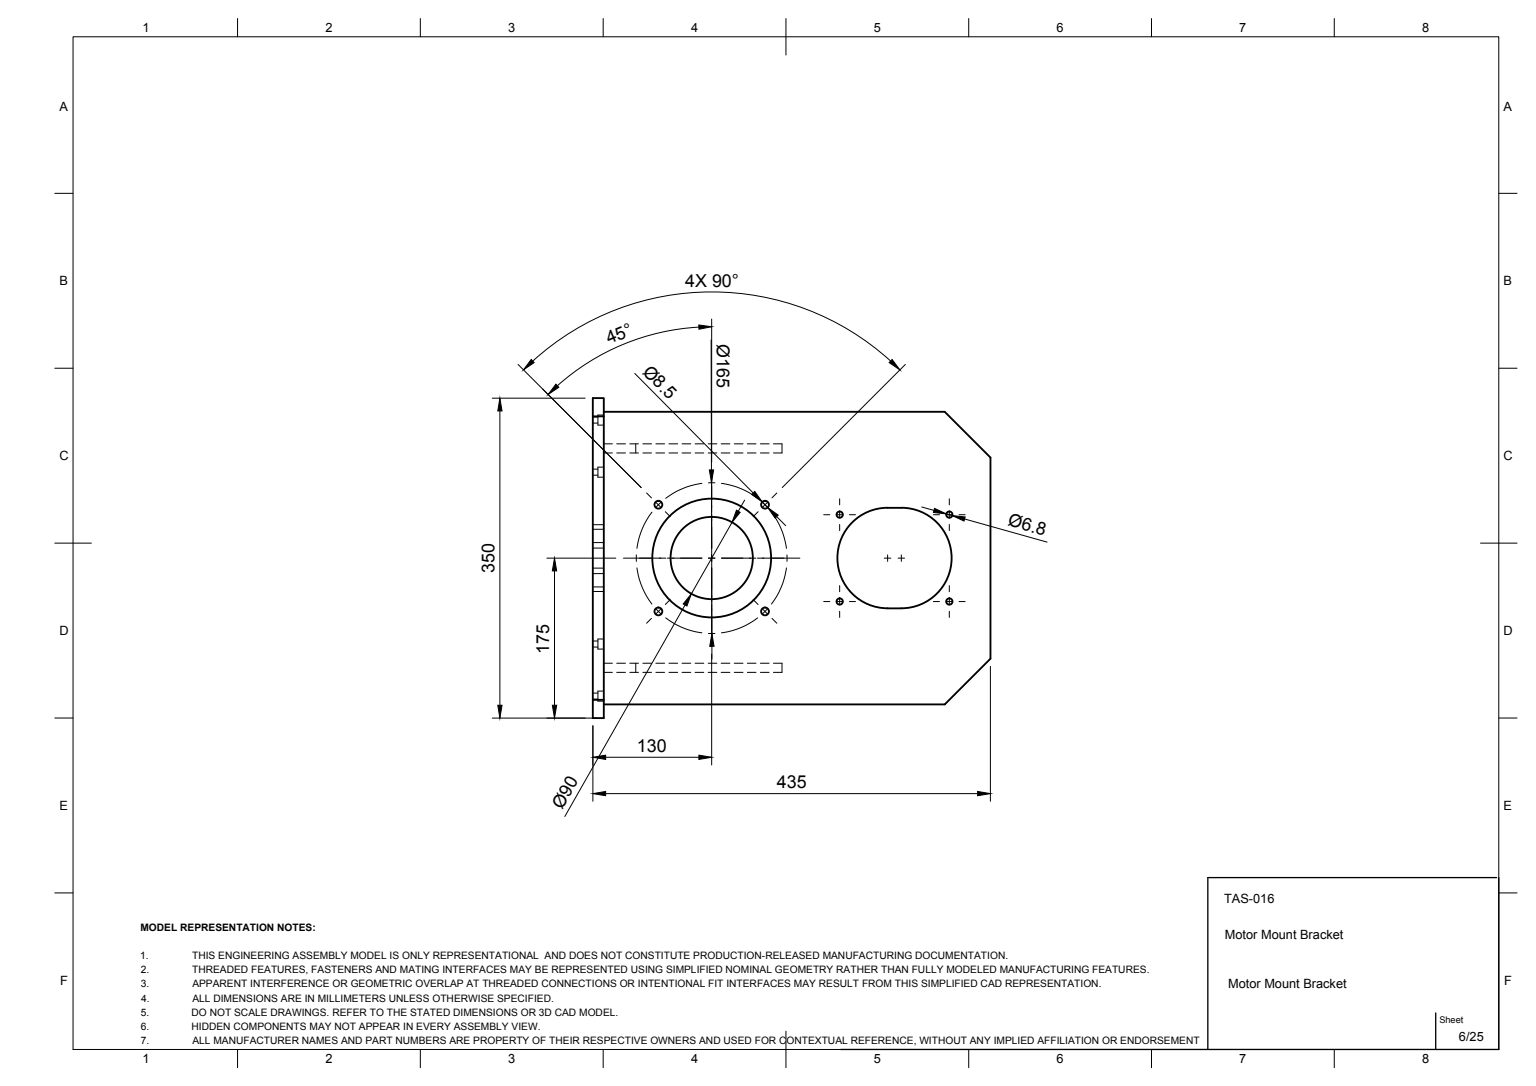
ISO-10303-21;
HEADER;
/* Generated by software containing ST-Developer
 * from STEP Tools, Inc. (www.steptools.com) 
 */

FILE_DESCRIPTION(
/* description */ ('STEP AP214'),
/* implementation_level */ '2;1');

FILE_NAME(
/* name */ 'Motor Mount Bracket.step',
/* time_stamp */ '2026-11-15T14:55:55-08:00',
/* author */ (''),
/* organization */ (''),
/* preprocessor_version */ 'ST-DEVELOPER v20.2',
/* originating_system */ 'Autodesk Translation Framework v15.17.0.0',
/* authorisation */ '');

FILE_SCHEMA (('AUTOMOTIVE_DESIGN { 1 0 10303 214 3 1 1 }'));
ENDSEC;

DATA;
#10=MECHANICAL_DESIGN_GEOMETRIC_PRESENTATION_REPRESENTATION('',(#947,#948,#949),#57079);
#887=SHAPE_REPRESENTATION_RELATIONSHIP('SRR','None',#57276,#916);
#916=ADVANCED_BREP_SHAPE_REPRESENTATION('',(#984,#985,#986),#57068);
#947=STYLED_ITEM('',(#57444),#984);
#948=STYLED_ITEM('',(#57444),#985);
#949=STYLED_ITEM('',(#57444),#986);
#984=MANIFOLD_SOLID_BREP('Body1',#24547);
#985=MANIFOLD_SOLID_BREP('Body2',#24548);
#986=MANIFOLD_SOLID_BREP('Body3',#24549);
#1195=FACE_BOUND('',#4460,.T.);
#1196=FACE_BOUND('',#4461,.T.);
#1197=FACE_BOUND('',#4462,.T.);
#1198=FACE_BOUND('',#4463,.T.);
#1199=FACE_BOUND('',#4464,.T.);
#1200=FACE_BOUND('',#4465,.T.);
#1201=FACE_BOUND('',#4466,.T.);
#1202=FACE_BOUND('',#4467,.T.);
#1203=FACE_BOUND('',#4468,.T.);
#1204=FACE_BOUND('',#4469,.T.);
#1205=FACE_BOUND('',#4470,.T.);
#1206=FACE_BOUND('',#4471,.T.);
#1207=FACE_BOUND('',#4472,.T.);
#1208=FACE_BOUND('',#4473,.T.);
#1209=FACE_BOUND('',#4474,.T.);
#1210=FACE_BOUND('',#4475,.T.);
#1211=FACE_BOUND('',#4476,.T.);
#1212=FACE_BOUND('',#4477,.T.);
#1213=FACE_BOUND('',#4478,.T.);
#1214=FACE_BOUND('',#4479,.T.);
#1215=FACE_BOUND('',#4480,.T.);
#1216=FACE_BOUND('',#4481,.T.);
#1217=FACE_BOUND('',#4486,.T.);
#1218=FACE_BOUND('',#4487,.T.);
#1219=FACE_BOUND('',#4488,.T.);
#1220=FACE_BOUND('',#4489,.T.);
#1221=FACE_BOUND('',#4490,.T.);
#1222=FACE_BOUND('',#4491,.T.);
#1223=FACE_BOUND('',#4492,.T.);
#1224=FACE_BOUND('',#4493,.T.);
#1225=FACE_BOUND('',#4494,.T.);
#1226=FACE_BOUND('',#4495,.T.);
#1227=FACE_BOUND('',#4497,.T.);
#1228=FACE_BOUND('',#4498,.T.);
#1229=FACE_BOUND('',#4499,.T.);
#1230=FACE_BOUND('',#4500,.T.);
#1231=FACE_BOUND('',#4501,.T.);
#1232=FACE_BOUND('',#4502,.T.);
#1233=FACE_BOUND('',#4503,.T.);
#1234=FACE_BOUND('',#4504,.T.);
#1235=FACE_BOUND('',#4505,.T.);
#1236=FACE_BOUND('',#4506,.T.);
#1237=FACE_BOUND('',#4508,.T.);
#1238=FACE_BOUND('',#4509,.T.);
#1239=FACE_BOUND('',#4510,.T.);
#1240=FACE_BOUND('',#4511,.T.);
#1241=FACE_BOUND('',#4512,.T.);
#1242=FACE_BOUND('',#4513,.T.);
#1243=FACE_BOUND('',#4514,.T.);
#1244=FACE_BOUND('',#4515,.T.);
#1245=FACE_BOUND('',#4516,.T.);
#1246=FACE_BOUND('',#4517,.T.);
#1247=FACE_BOUND('',#4518,.T.);
#1248=FACE_BOUND('',#4519,.T.);
#1249=FACE_BOUND('',#4520,.T.);
#1250=FACE_BOUND('',#4521,.T.);
#1251=FACE_BOUND('',#4522,.T.);
#1252=FACE_BOUND('',#4523,.T.);
#1253=FACE_BOUND('',#4524,.T.);
#1254=FACE_BOUND('',#4525,.T.);
#1255=FACE_BOUND('',#4526,.T.);
#1256=FACE_BOUND('',#4527,.T.);
#1257=FACE_BOUND('',#4528,.T.);
#1258=FACE_BOUND('',#4529,.T.);
#1259=FACE_BOUND('',#4530,.T.);
#1260=FACE_BOUND('',#4536,.T.);
#1261=FACE_BOUND('',#4538,.T.);
#1262=FACE_BOUND('',#4540,.T.);
#1263=FACE_BOUND('',#4542,.T.);
#1264=FACE_BOUND('',#4544,.T.);
#1265=FACE_BOUND('',#4546,.T.);
#1266=FACE_BOUND('',#4548,.T.);
#1267=FACE_BOUND('',#4550,.T.);
#1268=FACE_BOUND('',#4552,.T.);
#1269=FACE_BOUND('',#4554,.T.);
#1270=FACE_BOUND('',#4556,.T.);
#1271=FACE_BOUND('',#4558,.T.);
#1272=FACE_BOUND('',#4560,.T.);
#1273=FACE_BOUND('',#4562,.T.);
#1274=FACE_BOUND('',#4564,.T.);
#1275=FACE_BOUND('',#4566,.T.);
#1276=FACE_BOUND('',#4568,.T.);
#1680=PLANE('',#26069);
#1681=PLANE('',#26070);
#1682=PLANE('',#26071);
#1683=PLANE('',#26072);
#1684=PLANE('',#26073);
#1685=PLANE('',#26074);
#1686=PLANE('',#26075);
#1687=PLANE('',#26076);
#1688=PLANE('',#26077);
#1689=PLANE('',#26078);
#1690=PLANE('',#26079);
#1691=PLANE('',#26080);
#1692=PLANE('',#26081);
#1693=PLANE('',#26082);
#1694=PLANE('',#26230);
#1695=PLANE('',#26231);
#1696=PLANE('',#26232);
#1697=PLANE('',#26233);
#1698=PLANE('',#26234);
#1699=PLANE('',#26236);
#1700=PLANE('',#26238);
#1701=PLANE('',#26239);
#1702=PLANE('',#26240);
#1703=PLANE('',#26241);
#1704=PLANE('',#26242);
#1705=PLANE('',#26243);
#1706=PLANE('',#26244);
#1707=PLANE('',#26245);
#1708=PLANE('',#26246);
#1709=PLANE('',#26247);
#1710=PLANE('',#26248);
#1711=PLANE('',#26249);
#1712=PLANE('',#26250);
#1713=PLANE('',#26251);
#1714=PLANE('',#26252);
#1715=PLANE('',#26253);
#1716=PLANE('',#26254);
#1717=PLANE('',#26255);
#1718=PLANE('',#26256);
#1719=PLANE('',#26257);
#1720=PLANE('',#26258);
#1721=PLANE('',#26259);
#1722=PLANE('',#26260);
#1723=PLANE('',#26261);
#1724=PLANE('',#26262);
#1725=PLANE('',#26263);
#1726=PLANE('',#26265);
#1727=PLANE('',#26266);
#1728=PLANE('',#26267);
#1729=PLANE('',#26268);
#2826=FACE_OUTER_BOUND('',#4396,.T.);
#2827=FACE_OUTER_BOUND('',#4397,.T.);
#2828=FACE_OUTER_BOUND('',#4398,.T.);
#2829=FACE_OUTER_BOUND('',#4399,.T.);
#2830=FACE_OUTER_BOUND('',#4400,.T.);
#2831=FACE_OUTER_BOUND('',#4401,.T.);
#2832=FACE_OUTER_BOUND('',#4402,.T.);
#2833=FACE_OUTER_BOUND('',#4403,.T.);
#2834=FACE_OUTER_BOUND('',#4404,.T.);
#2835=FACE_OUTER_BOUND('',#4405,.T.);
#2836=FACE_OUTER_BOUND('',#4406,.T.);
#2837=FACE_OUTER_BOUND('',#4407,.T.);
#2838=FACE_OUTER_BOUND('',#4408,.T.);
#2839=FACE_OUTER_BOUND('',#4409,.T.);
#2840=FACE_OUTER_BOUND('',#4410,.T.);
#2841=FACE_OUTER_BOUND('',#4411,.T.);
#2842=FACE_OUTER_BOUND('',#4412,.T.);
#2843=FACE_OUTER_BOUND('',#4413,.T.);
#2844=FACE_OUTER_BOUND('',#4414,.T.);
#2845=FACE_OUTER_BOUND('',#4415,.T.);
#2846=FACE_OUTER_BOUND('',#4416,.T.);
#2847=FACE_OUTER_BOUND('',#4417,.T.);
#2848=FACE_OUTER_BOUND('',#4418,.T.);
#2849=FACE_OUTER_BOUND('',#4419,.T.);
#2850=FACE_OUTER_BOUND('',#4420,.T.);
#2851=FACE_OUTER_BOUND('',#4421,.T.);
#2852=FACE_OUTER_BOUND('',#4422,.T.);
#2853=FACE_OUTER_BOUND('',#4423,.T.);
#2854=FACE_OUTER_BOUND('',#4424,.T.);
#2855=FACE_OUTER_BOUND('',#4425,.T.);
#2856=FACE_OUTER_BOUND('',#4426,.T.);
#2857=FACE_OUTER_BOUND('',#4427,.T.);
#2858=FACE_OUTER_BOUND('',#4428,.T.);
#2859=FACE_OUTER_BOUND('',#4429,.T.);
#2860=FACE_OUTER_BOUND('',#4430,.T.);
#2861=FACE_OUTER_BOUND('',#4431,.T.);
#2862=FACE_OUTER_BOUND('',#4432,.T.);
#2863=FACE_OUTER_BOUND('',#4433,.T.);
#2864=FACE_OUTER_BOUND('',#4434,.T.);
#2865=FACE_OUTER_BOUND('',#4435,.T.);
#2866=FACE_OUTER_BOUND('',#4436,.T.);
#2867=FACE_OUTER_BOUND('',#4437,.T.);
#2868=FACE_OUTER_BOUND('',#4438,.T.);
#2869=FACE_OUTER_BOUND('',#4439,.T.);
#2870=FACE_OUTER_BOUND('',#4440,.T.);
#2871=FACE_OUTER_BOUND('',#4441,.T.);
#2872=FACE_OUTER_BOUND('',#4442,.T.);
#2873=FACE_OUTER_BOUND('',#4443,.T.);
#2874=FACE_OUTER_BOUND('',#4444,.T.);
#2875=FACE_OUTER_BOUND('',#4445,.T.);
#2876=FACE_OUTER_BOUND('',#4446,.T.);
#2877=FACE_OUTER_BOUND('',#4447,.T.);
#2878=FACE_OUTER_BOUND('',#4448,.T.);
#2879=FACE_OUTER_BOUND('',#4449,.T.);
#2880=FACE_OUTER_BOUND('',#4450,.T.);
#2881=FACE_OUTER_BOUND('',#4451,.T.);
#2882=FACE_OUTER_BOUND('',#4452,.T.);
#2883=FACE_OUTER_BOUND('',#4453,.T.);
#2884=FACE_OUTER_BOUND('',#4454,.T.);
#2885=FACE_OUTER_BOUND('',#4455,.T.);
#2886=FACE_OUTER_BOUND('',#4456,.T.);
#2887=FACE_OUTER_BOUND('',#4457,.T.);
#2888=FACE_OUTER_BOUND('',#4458,.T.);
#2889=FACE_OUTER_BOUND('',#4459,.T.);
#2890=FACE_OUTER_BOUND('',#4482,.T.);
#2891=FACE_OUTER_BOUND('',#4483,.T.);
#2892=FACE_OUTER_BOUND('',#4484,.T.);
#2893=FACE_OUTER_BOUND('',#4485,.T.);
#2894=FACE_OUTER_BOUND('',#4496,.T.);
#2895=FACE_OUTER_BOUND('',#4507,.T.);
#2896=FACE_OUTER_BOUND('',#4531,.T.);
#2897=FACE_OUTER_BOUND('',#4532,.T.);
#2898=FACE_OUTER_BOUND('',#4533,.T.);
#2899=FACE_OUTER_BOUND('',#4534,.T.);
#2900=FACE_OUTER_BOUND('',#4535,.T.);
#2901=FACE_OUTER_BOUND('',#4537,.T.);
#2902=FACE_OUTER_BOUND('',#4539,.T.);
#2903=FACE_OUTER_BOUND('',#4541,.T.);
#2904=FACE_OUTER_BOUND('',#4543,.T.);
#2905=FACE_OUTER_BOUND('',#4545,.T.);
#2906=FACE_OUTER_BOUND('',#4547,.T.);
#2907=FACE_OUTER_BOUND('',#4549,.T.);
#2908=FACE_OUTER_BOUND('',#4551,.T.);
#2909=FACE_OUTER_BOUND('',#4553,.T.);
#2910=FACE_OUTER_BOUND('',#4555,.T.);
#2911=FACE_OUTER_BOUND('',#4557,.T.);
#2912=FACE_OUTER_BOUND('',#4559,.T.);
#2913=FACE_OUTER_BOUND('',#4561,.T.);
#2914=FACE_OUTER_BOUND('',#4563,.T.);
#2915=FACE_OUTER_BOUND('',#4565,.T.);
#2916=FACE_OUTER_BOUND('',#4567,.T.);
#2917=FACE_OUTER_BOUND('',#4569,.T.);
#2918=FACE_OUTER_BOUND('',#4570,.T.);
#2919=FACE_OUTER_BOUND('',#4571,.T.);
#2920=FACE_OUTER_BOUND('',#4572,.T.);
#2921=FACE_OUTER_BOUND('',#4573,.T.);
#2922=FACE_OUTER_BOUND('',#4574,.T.);
#2923=FACE_OUTER_BOUND('',#4575,.T.);
#2924=FACE_OUTER_BOUND('',#4576,.T.);
#2925=FACE_OUTER_BOUND('',#4577,.T.);
#4396=EDGE_LOOP('',(#19072,#19073,#19074,#19075));
#4397=EDGE_LOOP('',(#19076,#19077,#19078,#19079));
#4398=EDGE_LOOP('',(#19080,#19081,#19082,#19083));
#4399=EDGE_LOOP('',(#19084,#19085,#19086,#19087));
#4400=EDGE_LOOP('',(#19088,#19089,#19090,#19091));
#4401=EDGE_LOOP('',(#19092,#19093,#19094,#19095,#19096));
#4402=EDGE_LOOP('',(#19097,#19098,#19099,#19100,#19101));
#4403=EDGE_LOOP('',(#19102,#19103,#19104,#19105));
#4404=EDGE_LOOP('',(#19106,#19107,#19108,#19109));
#4405=EDGE_LOOP('',(#19110,#19111,#19112,#19113));
#4406=EDGE_LOOP('',(#19114,#19115,#19116,#19117));
#4407=EDGE_LOOP('',(#19118,#19119,#19120,#19121));
#4408=EDGE_LOOP('',(#19122,#19123,#19124,#19125,#19126));
#4409=EDGE_LOOP('',(#19127,#19128,#19129,#19130,#19131));
#4410=EDGE_LOOP('',(#19132,#19133,#19134,#19135));
#4411=EDGE_LOOP('',(#19136,#19137,#19138,#19139));
#4412=EDGE_LOOP('',(#19140,#19141,#19142,#19143));
#4413=EDGE_LOOP('',(#19144,#19145,#19146,#19147));
#4414=EDGE_LOOP('',(#19148,#19149,#19150,#19151));
#4415=EDGE_LOOP('',(#19152,#19153,#19154,#19155));
#4416=EDGE_LOOP('',(#19156,#19157,#19158,#19159));
#4417=EDGE_LOOP('',(#19160,#19161,#19162,#19163));
#4418=EDGE_LOOP('',(#19164,#19165,#19166,#19167));
#4419=EDGE_LOOP('',(#19168,#19169,#19170,#19171));
#4420=EDGE_LOOP('',(#19172,#19173,#19174,#19175));
#4421=EDGE_LOOP('',(#19176,#19177,#19178,#19179));
#4422=EDGE_LOOP('',(#19180,#19181,#19182,#19183));
#4423=EDGE_LOOP('',(#19184,#19185,#19186,#19187));
#4424=EDGE_LOOP('',(#19188,#19189,#19190,#19191));
#4425=EDGE_LOOP('',(#19192,#19193,#19194,#19195));
#4426=EDGE_LOOP('',(#19196,#19197,#19198,#19199));
#4427=EDGE_LOOP('',(#19200,#19201,#19202,#19203));
#4428=EDGE_LOOP('',(#19204,#19205,#19206,#19207));
#4429=EDGE_LOOP('',(#19208,#19209,#19210,#19211));
#4430=EDGE_LOOP('',(#19212,#19213,#19214,#19215));
#4431=EDGE_LOOP('',(#19216,#19217,#19218,#19219));
#4432=EDGE_LOOP('',(#19220,#19221,#19222,#19223));
#4433=EDGE_LOOP('',(#19224,#19225,#19226,#19227));
#4434=EDGE_LOOP('',(#19228,#19229,#19230,#19231));
#4435=EDGE_LOOP('',(#19232,#19233,#19234,#19235));
#4436=EDGE_LOOP('',(#19236,#19237,#19238,#19239));
#4437=EDGE_LOOP('',(#19240,#19241,#19242,#19243));
#4438=EDGE_LOOP('',(#19244,#19245,#19246,#19247));
#4439=EDGE_LOOP('',(#19248,#19249,#19250,#19251));
#4440=EDGE_LOOP('',(#19252,#19253,#19254,#19255));
#4441=EDGE_LOOP('',(#19256,#19257,#19258,#19259));
#4442=EDGE_LOOP('',(#19260,#19261,#19262,#19263));
#4443=EDGE_LOOP('',(#19264,#19265,#19266,#19267));
#4444=EDGE_LOOP('',(#19268,#19269,#19270,#19271));
#4445=EDGE_LOOP('',(#19272,#19273,#19274,#19275));
#4446=EDGE_LOOP('',(#19276,#19277,#19278,#19279));
#4447=EDGE_LOOP('',(#19280,#19281,#19282,#19283));
#4448=EDGE_LOOP('',(#19284,#19285,#19286,#19287));
#4449=EDGE_LOOP('',(#19288,#19289,#19290,#19291));
#4450=EDGE_LOOP('',(#19292,#19293,#19294,#19295));
#4451=EDGE_LOOP('',(#19296,#19297,#19298,#19299));
#4452=EDGE_LOOP('',(#19300,#19301,#19302,#19303));
#4453=EDGE_LOOP('',(#19304,#19305,#19306,#19307));
#4454=EDGE_LOOP('',(#19308,#19309,#19310,#19311));
#4455=EDGE_LOOP('',(#19312,#19313,#19314,#19315));
#4456=EDGE_LOOP('',(#19316,#19317,#19318,#19319));
#4457=EDGE_LOOP('',(#19320,#19321,#19322,#19323));
#4458=EDGE_LOOP('',(#19324,#19325,#19326,#19327));
#4459=EDGE_LOOP('',(#19328,#19329,#19330,#19331,#19332,#19333,#19334,#19335));
#4460=EDGE_LOOP('',(#19336));
#4461=EDGE_LOOP('',(#19337));
#4462=EDGE_LOOP('',(#19338));
#4463=EDGE_LOOP('',(#19339));
#4464=EDGE_LOOP('',(#19340));
#4465=EDGE_LOOP('',(#19341));
#4466=EDGE_LOOP('',(#19342));
#4467=EDGE_LOOP('',(#19343));
#4468=EDGE_LOOP('',(#19344));
#4469=EDGE_LOOP('',(#19345));
#4470=EDGE_LOOP('',(#19346));
#4471=EDGE_LOOP('',(#19347));
#4472=EDGE_LOOP('',(#19348));
#4473=EDGE_LOOP('',(#19349));
#4474=EDGE_LOOP('',(#19350));
#4475=EDGE_LOOP('',(#19351));
#4476=EDGE_LOOP('',(#19352));
#4477=EDGE_LOOP('',(#19353));
#4478=EDGE_LOOP('',(#19354));
#4479=EDGE_LOOP('',(#19355));
#4480=EDGE_LOOP('',(#19356));
#4481=EDGE_LOOP('',(#19357));
#4482=EDGE_LOOP('',(#19358,#19359,#19360,#19361));
#4483=EDGE_LOOP('',(#19362,#19363,#19364,#19365));
#4484=EDGE_LOOP('',(#19366,#19367,#19368,#19369));
#4485=EDGE_LOOP('',(#19370,#19371,#19372,#19373,#19374,#19375));
#4486=EDGE_LOOP('',(#19376));
#4487=EDGE_LOOP('',(#19377));
#4488=EDGE_LOOP('',(#19378));
#4489=EDGE_LOOP('',(#19379));
#4490=EDGE_LOOP('',(#19380,#19381,#19382,#19383));
#4491=EDGE_LOOP('',(#19384));
#4492=EDGE_LOOP('',(#19385));
#4493=EDGE_LOOP('',(#19386));
#4494=EDGE_LOOP('',(#19387));
#4495=EDGE_LOOP('',(#19388));
#4496=EDGE_LOOP('',(#19389,#19390,#19391,#19392,#19393,#19394));
#4497=EDGE_LOOP('',(#19395,#19396,#19397,#19398));
#4498=EDGE_LOOP('',(#19399));
#4499=EDGE_LOOP('',(#19400));
#4500=EDGE_LOOP('',(#19401));
#4501=EDGE_LOOP('',(#19402));
#4502=EDGE_LOOP('',(#19403));
#4503=EDGE_LOOP('',(#19404));
#4504=EDGE_LOOP('',(#19405));
#4505=EDGE_LOOP('',(#19406));
#4506=EDGE_LOOP('',(#19407));
#4507=EDGE_LOOP('',(#19408,#19409,#19410,#19411,#19412,#19413,#19414,#19415));
#4508=EDGE_LOOP('',(#19416,#19417,#19418,#19419));
#4509=EDGE_LOOP('',(#19420));
#4510=EDGE_LOOP('',(#19421));
#4511=EDGE_LOOP('',(#19422));
#4512=EDGE_LOOP('',(#19423));
#4513=EDGE_LOOP('',(#19424));
#4514=EDGE_LOOP('',(#19425));
#4515=EDGE_LOOP('',(#19426));
#4516=EDGE_LOOP('',(#19427));
#4517=EDGE_LOOP('',(#19428));
#4518=EDGE_LOOP('',(#19429));
#4519=EDGE_LOOP('',(#19430));
#4520=EDGE_LOOP('',(#19431));
#4521=EDGE_LOOP('',(#19432));
#4522=EDGE_LOOP('',(#19433));
#4523=EDGE_LOOP('',(#19434));
#4524=EDGE_LOOP('',(#19435));
#4525=EDGE_LOOP('',(#19436));
#4526=EDGE_LOOP('',(#19437));
#4527=EDGE_LOOP('',(#19438));
#4528=EDGE_LOOP('',(#19439));
#4529=EDGE_LOOP('',(#19440));
#4530=EDGE_LOOP('',(#19441));
#4531=EDGE_LOOP('',(#19442,#19443,#19444,#19445));
#4532=EDGE_LOOP('',(#19446,#19447,#19448,#19449));
#4533=EDGE_LOOP('',(#19450,#19451,#19452,#19453));
#4534=EDGE_LOOP('',(#19454,#19455,#19456,#19457));
#4535=EDGE_LOOP('',(#19458));
#4536=EDGE_LOOP('',(#19459));
#4537=EDGE_LOOP('',(#19460));
#4538=EDGE_LOOP('',(#19461));
#4539=EDGE_LOOP('',(#19462));
#4540=EDGE_LOOP('',(#19463));
#4541=EDGE_LOOP('',(#19464));
#4542=EDGE_LOOP('',(#19465));
#4543=EDGE_LOOP('',(#19466));
#4544=EDGE_LOOP('',(#19467));
#4545=EDGE_LOOP('',(#19468));
#4546=EDGE_LOOP('',(#19469));
#4547=EDGE_LOOP('',(#19470));
#4548=EDGE_LOOP('',(#19471));
#4549=EDGE_LOOP('',(#19472));
#4550=EDGE_LOOP('',(#19473));
#4551=EDGE_LOOP('',(#19474));
#4552=EDGE_LOOP('',(#19475));
#4553=EDGE_LOOP('',(#19476));
#4554=EDGE_LOOP('',(#19477));
#4555=EDGE_LOOP('',(#19478));
#4556=EDGE_LOOP('',(#19479));
#4557=EDGE_LOOP('',(#19480));
#4558=EDGE_LOOP('',(#19481));
#4559=EDGE_LOOP('',(#19482));
#4560=EDGE_LOOP('',(#19483));
#4561=EDGE_LOOP('',(#19484));
#4562=EDGE_LOOP('',(#19485));
#4563=EDGE_LOOP('',(#19486));
#4564=EDGE_LOOP('',(#19487));
#4565=EDGE_LOOP('',(#19488));
#4566=EDGE_LOOP('',(#19489));
#4567=EDGE_LOOP('',(#19490));
#4568=EDGE_LOOP('',(#19491));
#4569=EDGE_LOOP('',(#19492,#19493,#19494,#19495));
#4570=EDGE_LOOP('',(#19496,#19497,#19498,#19499));
#4571=EDGE_LOOP('',(#19500,#19501,#19502,#19503));
#4572=EDGE_LOOP('',(#19504,#19505,#19506,#19507));
#4573=EDGE_LOOP('',(#19508,#19509,#19510,#19511));
#4574=EDGE_LOOP('',(#19512,#19513,#19514,#19515));
#4575=EDGE_LOOP('',(#19516,#19517,#19518,#19519));
#4576=EDGE_LOOP('',(#19520,#19521,#19522,#19523));
#4577=EDGE_LOOP('',(#19524,#19525,#19526,#19527));
#6035=LINE('',#52991,#8002);
#6036=LINE('',#52993,#8003);
#6037=LINE('',#52995,#8004);
#6038=LINE('',#52996,#8005);
#6039=LINE('',#52999,#8006);
#6040=LINE('',#53001,#8007);
#6041=LINE('',#53002,#8008);
#6042=LINE('',#53005,#8009);
#6043=LINE('',#53007,#8010);
#6044=LINE('',#53008,#8011);
#6045=LINE('',#53011,#8012);
#6046=LINE('',#53013,#8013);
#6047=LINE('',#53014,#8014);
#6048=LINE('',#53016,#8015);
#6049=LINE('',#53017,#8016);
#6050=LINE('',#53023,#8017);
#6051=LINE('',#53025,#8018);
#6052=LINE('',#53027,#8019);
#6053=LINE('',#53028,#8020);
#6054=LINE('',#53031,#8021);
#6055=LINE('',#53033,#8022);
#6056=LINE('',#53034,#8023);
#6057=LINE('',#53037,#8024);
#6058=LINE('',#53039,#8025);
#6059=LINE('',#53040,#8026);
#6060=LINE('',#53043,#8027);
#6061=LINE('',#53045,#8028);
#6062=LINE('',#53046,#8029);
#6063=LINE('',#53048,#8030);
#6064=LINE('',#53049,#8031);
#6065=LINE('',#53057,#8032);
#6066=LINE('',#53060,#8033);
#6067=LINE('',#53065,#8034);
#6068=LINE('',#53071,#8035);
#6069=LINE('',#53077,#8036);
#6070=LINE('',#53083,#8037);
#6071=LINE('',#53089,#8038);
#6072=LINE('',#53095,#8039);
#6073=LINE('',#53101,#8040);
#6074=LINE('',#53107,#8041);
#6075=LINE('',#53113,#8042);
#6076=LINE('',#53119,#8043);
#6077=LINE('',#53125,#8044);
#6078=LINE('',#53131,#8045);
#6079=LINE('',#53137,#8046);
#6080=LINE('',#53143,#8047);
#6081=LINE('',#53149,#8048);
#6082=LINE('',#53155,#8049);
#6083=LINE('',#53161,#8050);
#6084=LINE('',#53167,#8051);
#6085=LINE('',#53173,#8052);
#6086=LINE('',#53179,#8053);
#6087=LINE('',#53185,#8054);
#6088=LINE('',#53191,#8055);
#6089=LINE('',#53197,#8056);
#6090=LINE('',#53203,#8057);
#6091=LINE('',#53209,#8058);
#6092=LINE('',#53215,#8059);
#6093=LINE('',#53221,#8060);
#6094=LINE('',#53227,#8061);
#6095=LINE('',#53233,#8062);
#6096=LINE('',#53239,#8063);
#6097=LINE('',#53245,#8064);
#6098=LINE('',#53251,#8065);
#6099=LINE('',#53257,#8066);
#6100=LINE('',#53263,#8067);
#6101=LINE('',#53269,#8068);
#6102=LINE('',#53275,#8069);
#6103=LINE('',#53281,#8070);
#6104=LINE('',#53287,#8071);
#6105=LINE('',#53293,#8072);
#6106=LINE('',#53299,#8073);
#6107=LINE('',#53305,#8074);
#6108=LINE('',#53311,#8075);
#6109=LINE('',#53317,#8076);
#6110=LINE('',#53323,#8077);
#6111=LINE('',#53329,#8078);
#6112=LINE('',#53335,#8079);
#6113=LINE('',#53341,#8080);
#6114=LINE('',#53347,#8081);
#6115=LINE('',#53352,#8082);
#6116=LINE('',#53354,#8083);
#6117=LINE('',#53356,#8084);
#6118=LINE('',#53358,#8085);
#6119=LINE('',#53360,#8086);
#6120=LINE('',#53362,#8087);
#6121=LINE('',#53364,#8088);
#6122=LINE('',#53365,#8089);
#6123=LINE('',#53369,#8090);
#6124=LINE('',#53371,#8091);
#6125=LINE('',#53373,#8092);
#6126=LINE('',#53374,#8093);
#6127=LINE('',#53378,#8094);
#6128=LINE('',#53380,#8095);
#6129=LINE('',#53382,#8096);
#6130=LINE('',#53383,#8097);
#6131=LINE('',#53387,#8098);
#6132=LINE('',#53389,#8099);
#6133=LINE('',#53391,#8100);
#6134=LINE('',#53392,#8101);
#6135=LINE('',#53394,#8102);
#6136=LINE('',#53395,#8103);
#6137=LINE('',#53396,#8104);
#6138=LINE('',#53398,#8105);
#6139=LINE('',#53400,#8106);
#6140=LINE('',#53403,#8107);
#6141=LINE('',#53404,#8108);
#6142=LINE('',#53405,#8109);
#6143=LINE('',#53407,#8110);
#6144=LINE('',#53410,#8111);
#6145=LINE('',#53414,#8112);
#6146=LINE('',#53416,#8113);
#6147=LINE('',#53418,#8114);
#6148=LINE('',#53420,#8115);
#6149=LINE('',#53422,#8116);
#6150=LINE('',#53424,#8117);
#6151=LINE('',#53426,#8118);
#6152=LINE('',#53427,#8119);
#6153=LINE('',#53429,#8120);
#6154=LINE('',#53430,#8121);
#6155=LINE('',#53432,#8122);
#6156=LINE('',#53433,#8123);
#6157=LINE('',#53435,#8124);
#6158=LINE('',#53436,#8125);
#6159=LINE('',#53438,#8126);
#6160=LINE('',#53439,#8127);
#6161=LINE('',#53460,#8128);
#6162=LINE('',#53462,#8129);
#8002=VECTOR('',#30635,1000.);
#8003=VECTOR('',#30636,1000.);
#8004=VECTOR('',#30637,1000.);
#8005=VECTOR('',#30638,1000.);
#8006=VECTOR('',#30641,1000.);
#8007=VECTOR('',#30642,1000.);
#8008=VECTOR('',#30643,1000.);
#8009=VECTOR('',#30646,1000.);
#8010=VECTOR('',#30647,1000.);
#8011=VECTOR('',#30648,1000.);
#8012=VECTOR('',#30651,1000.);
#8013=VECTOR('',#30652,1000.);
#8014=VECTOR('',#30653,1000.);
#8015=VECTOR('',#30656,1000.);
#8016=VECTOR('',#30657,1000.);
#8017=VECTOR('',#30664,1000.);
#8018=VECTOR('',#30665,1000.);
#8019=VECTOR('',#30666,1000.);
#8020=VECTOR('',#30667,1000.);
#8021=VECTOR('',#30670,1000.);
#8022=VECTOR('',#30671,1000.);
#8023=VECTOR('',#30672,1000.);
#8024=VECTOR('',#30675,1000.);
#8025=VECTOR('',#30676,1000.);
#8026=VECTOR('',#30677,1000.);
#8027=VECTOR('',#30680,1000.);
#8028=VECTOR('',#30681,1000.);
#8029=VECTOR('',#30682,1000.);
#8030=VECTOR('',#30685,1000.);
#8031=VECTOR('',#30686,1000.);
#8032=VECTOR('',#30695,1000.);
#8033=VECTOR('',#30698,1000.);
#8034=VECTOR('',#30703,3.39999999999999);
#8035=VECTOR('',#30710,3.4);
#8036=VECTOR('',#30717,3.4);
#8037=VECTOR('',#30724,3.39999999999999);
#8038=VECTOR('',#30731,4.24999999999998);
#8039=VECTOR('',#30738,4.24999999999998);
#8040=VECTOR('',#30745,4.24999999999998);
#8041=VECTOR('',#30752,4.24999999999998);
#8042=VECTOR('',#30759,45.);
#8043=VECTOR('',#30766,65.);
#8044=VECTOR('',#30773,2.99999999999999);
#8045=VECTOR('',#30780,2.99999999999999);
#8046=VECTOR('',#30787,2.5);
#8047=VECTOR('',#30794,2.5);
#8048=VECTOR('',#30801,2.5);
#8049=VECTOR('',#30808,2.5);
#8050=VECTOR('',#30815,5.50000000000001);
#8051=VECTOR('',#30822,3.30000000000004);
#8052=VECTOR('',#30829,5.50000000000001);
#8053=VECTOR('',#30836,3.30000000000004);
#8054=VECTOR('',#30843,5.50000000000001);
#8055=VECTOR('',#30850,3.30000000000004);
#8056=VECTOR('',#30857,5.50000000000001);
#8057=VECTOR('',#30864,3.30000000000004);
#8058=VECTOR('',#30871,5.50000000000001);
#8059=VECTOR('',#30878,3.30000000000004);
#8060=VECTOR('',#30885,5.50000000000001);
#8061=VECTOR('',#30892,3.30000000000004);
#8062=VECTOR('',#30899,5.49999999999999);
#8063=VECTOR('',#30906,3.30000000000004);
#8064=VECTOR('',#30913,5.50000000000001);
#8065=VECTOR('',#30920,3.30000000000004);
#8066=VECTOR('',#30927,5.50000000000001);
#8067=VECTOR('',#30934,3.30000000000004);
#8068=VECTOR('',#30941,5.50000000000001);
#8069=VECTOR('',#30948,3.30000000000004);
#8070=VECTOR('',#30955,5.50000000000001);
#8071=VECTOR('',#30962,3.30000000000004);
#8072=VECTOR('',#30969,5.50000000000001);
#8073=VECTOR('',#30976,3.30000000000004);
#8074=VECTOR('',#30983,5.50000000000001);
#8075=VECTOR('',#30990,3.30000000000004);
#8076=VECTOR('',#30997,5.50000000000001);
#8077=VECTOR('',#31004,3.30000000000004);
#8078=VECTOR('',#31011,5.49999999999999);
#8079=VECTOR('',#31018,3.30000000000004);
#8080=VECTOR('',#31025,5.50000000000001);
#8081=VECTOR('',#31032,3.30000000000004);
#8082=VECTOR('',#31037,1000.);
#8083=VECTOR('',#31038,1000.);
#8084=VECTOR('',#31039,1000.);
#8085=VECTOR('',#31040,1000.);
#8086=VECTOR('',#31041,1000.);
#8087=VECTOR('',#31042,1000.);
#8088=VECTOR('',#31043,1000.);
#8089=VECTOR('',#31044,1000.);
#8090=VECTOR('',#31047,1000.);
#8091=VECTOR('',#31048,1000.);
#8092=VECTOR('',#31049,1000.);
#8093=VECTOR('',#31050,1000.);
#8094=VECTOR('',#31053,1000.);
#8095=VECTOR('',#31054,1000.);
#8096=VECTOR('',#31055,1000.);
#8097=VECTOR('',#31056,1000.);
#8098=VECTOR('',#31059,1000.);
#8099=VECTOR('',#31060,1000.);
#8100=VECTOR('',#31061,1000.);
#8101=VECTOR('',#31062,1000.);
#8102=VECTOR('',#31065,1000.);
#8103=VECTOR('',#31066,1000.);
#8104=VECTOR('',#31067,1000.);
#8105=VECTOR('',#31068,1000.);
#8106=VECTOR('',#31069,1000.);
#8107=VECTOR('',#31074,1000.);
#8108=VECTOR('',#31075,1000.);
#8109=VECTOR('',#31076,1000.);
#8110=VECTOR('',#31077,1000.);
#8111=VECTOR('',#31080,1000.);
#8112=VECTOR('',#31083,1000.);
#8113=VECTOR('',#31084,1000.);
#8114=VECTOR('',#31085,1000.);
#8115=VECTOR('',#31086,1000.);
#8116=VECTOR('',#31087,1000.);
#8117=VECTOR('',#31088,1000.);
#8118=VECTOR('',#31089,1000.);
#8119=VECTOR('',#31090,1000.);
#8120=VECTOR('',#31093,1000.);
#8121=VECTOR('',#31094,1000.);
#8122=VECTOR('',#31097,1000.);
#8123=VECTOR('',#31098,1000.);
#8124=VECTOR('',#31101,1000.);
#8125=VECTOR('',#31102,1000.);
#8126=VECTOR('',#31105,1000.);
#8127=VECTOR('',#31106,1000.);
#8128=VECTOR('',#31147,1000.);
#8129=VECTOR('',#31150,1000.);
#9708=CIRCLE('',#26084,55.);
#9709=CIRCLE('',#26085,55.);
#9710=CIRCLE('',#26087,3.39999999999999);
#9711=CIRCLE('',#26088,3.4);
#9712=CIRCLE('',#26090,3.4);
#9713=CIRCLE('',#26091,3.4);
#9714=CIRCLE('',#26093,3.4);
#9715=CIRCLE('',#26094,3.4);
#9716=CIRCLE('',#26096,3.39999999999999);
#9717=CIRCLE('',#26097,3.4);
#9718=CIRCLE('',#26099,4.24999999999998);
#9719=CIRCLE('',#26100,4.24999999999998);
#9720=CIRCLE('',#26102,4.24999999999998);
#9721=CIRCLE('',#26103,4.24999999999998);
#9722=CIRCLE('',#26105,4.24999999999998);
#9723=CIRCLE('',#26106,4.24999999999998);
#9724=CIRCLE('',#26108,4.24999999999998);
#9725=CIRCLE('',#26109,4.24999999999998);
#9726=CIRCLE('',#26111,45.);
#9727=CIRCLE('',#26112,45.);
#9728=CIRCLE('',#26114,65.);
#9729=CIRCLE('',#26115,65.);
#9730=CIRCLE('',#26117,2.99999999999999);
#9731=CIRCLE('',#26118,2.99999999999999);
#9732=CIRCLE('',#26120,2.99999999999999);
#9733=CIRCLE('',#26121,2.99999999999999);
#9734=CIRCLE('',#26123,2.5);
#9735=CIRCLE('',#26124,2.5);
#9736=CIRCLE('',#26126,2.5);
#9737=CIRCLE('',#26127,2.5);
#9738=CIRCLE('',#26129,2.5);
#9739=CIRCLE('',#26130,2.5);
#9740=CIRCLE('',#26132,2.5);
#9741=CIRCLE('',#26133,2.5);
#9742=CIRCLE('',#26135,5.50000000000001);
#9743=CIRCLE('',#26136,5.50000000000001);
#9744=CIRCLE('',#26138,3.30000000000008);
#9745=CIRCLE('',#26139,3.3);
#9746=CIRCLE('',#26141,5.50000000000001);
#9747=CIRCLE('',#26142,5.50000000000001);
#9748=CIRCLE('',#26144,3.30000000000008);
#9749=CIRCLE('',#26145,3.3);
#9750=CIRCLE('',#26147,5.50000000000001);
#9751=CIRCLE('',#26148,5.50000000000001);
#9752=CIRCLE('',#26150,3.30000000000008);
#9753=CIRCLE('',#26151,3.3);
#9754=CIRCLE('',#26153,5.50000000000001);
#9755=CIRCLE('',#26154,5.50000000000001);
#9756=CIRCLE('',#26156,3.30000000000008);
#9757=CIRCLE('',#26157,3.3);
#9758=CIRCLE('',#26159,5.50000000000001);
#9759=CIRCLE('',#26160,5.50000000000001);
#9760=CIRCLE('',#26162,3.30000000000008);
#9761=CIRCLE('',#26163,3.3);
#9762=CIRCLE('',#26165,5.50000000000001);
#9763=CIRCLE('',#26166,5.50000000000001);
#9764=CIRCLE('',#26168,3.30000000000008);
#9765=CIRCLE('',#26169,3.3);
#9766=CIRCLE('',#26171,5.49999999999999);
#9767=CIRCLE('',#26172,5.49999999999999);
#9768=CIRCLE('',#26174,3.30000000000008);
#9769=CIRCLE('',#26175,3.3);
#9770=CIRCLE('',#26177,5.50000000000001);
#9771=CIRCLE('',#26178,5.50000000000001);
#9772=CIRCLE('',#26180,3.30000000000008);
#9773=CIRCLE('',#26181,3.3);
#9774=CIRCLE('',#26183,5.50000000000001);
#9775=CIRCLE('',#26184,5.50000000000001);
#9776=CIRCLE('',#26186,3.30000000000008);
#9777=CIRCLE('',#26187,3.3);
#9778=CIRCLE('',#26189,5.50000000000001);
#9779=CIRCLE('',#26190,5.50000000000001);
#9780=CIRCLE('',#26192,3.30000000000008);
#9781=CIRCLE('',#26193,3.3);
#9782=CIRCLE('',#26195,5.50000000000001);
#9783=CIRCLE('',#26196,5.50000000000001);
#9784=CIRCLE('',#26198,3.30000000000008);
#9785=CIRCLE('',#26199,3.3);
#9786=CIRCLE('',#26201,5.50000000000001);
#9787=CIRCLE('',#26202,5.50000000000001);
#9788=CIRCLE('',#26204,3.30000000000008);
#9789=CIRCLE('',#26205,3.3);
#9790=CIRCLE('',#26207,5.50000000000001);
#9791=CIRCLE('',#26208,5.50000000000001);
#9792=CIRCLE('',#26210,3.30000000000008);
#9793=CIRCLE('',#26211,3.3);
#9794=CIRCLE('',#26213,5.50000000000001);
#9795=CIRCLE('',#26214,5.50000000000001);
#9796=CIRCLE('',#26216,3.30000000000008);
#9797=CIRCLE('',#26217,3.3);
#9798=CIRCLE('',#26219,5.49999999999999);
#9799=CIRCLE('',#26220,5.49999999999999);
#9800=CIRCLE('',#26222,3.30000000000008);
#9801=CIRCLE('',#26223,3.3);
#9802=CIRCLE('',#26225,5.50000000000001);
#9803=CIRCLE('',#26226,5.50000000000001);
#9804=CIRCLE('',#26228,3.30000000000008);
#9805=CIRCLE('',#26229,3.3);
#9806=CIRCLE('',#26235,55.);
#9807=CIRCLE('',#26237,55.);
#11289=VERTEX_POINT('',#52989);
#11290=VERTEX_POINT('',#52990);
#11291=VERTEX_POINT('',#52992);
#11292=VERTEX_POINT('',#52994);
#11293=VERTEX_POINT('',#52998);
#11294=VERTEX_POINT('',#53000);
#11295=VERTEX_POINT('',#53004);
#11296=VERTEX_POINT('',#53006);
#11297=VERTEX_POINT('',#53010);
#11298=VERTEX_POINT('',#53012);
#11299=VERTEX_POINT('',#53021);
#11300=VERTEX_POINT('',#53022);
#11301=VERTEX_POINT('',#53024);
#11302=VERTEX_POINT('',#53026);
#11303=VERTEX_POINT('',#53030);
#11304=VERTEX_POINT('',#53032);
#11305=VERTEX_POINT('',#53036);
#11306=VERTEX_POINT('',#53038);
#11307=VERTEX_POINT('',#53042);
#11308=VERTEX_POINT('',#53044);
#11309=VERTEX_POINT('',#53053);
#11310=VERTEX_POINT('',#53054);
#11311=VERTEX_POINT('',#53056);
#11312=VERTEX_POINT('',#53058);
#11313=VERTEX_POINT('',#53062);
#11314=VERTEX_POINT('',#53064);
#11315=VERTEX_POINT('',#53068);
#11316=VERTEX_POINT('',#53070);
#11317=VERTEX_POINT('',#53074);
#11318=VERTEX_POINT('',#53076);
#11319=VERTEX_POINT('',#53080);
#11320=VERTEX_POINT('',#53082);
#11321=VERTEX_POINT('',#53086);
#11322=VERTEX_POINT('',#53088);
#11323=VERTEX_POINT('',#53092);
#11324=VERTEX_POINT('',#53094);
#11325=VERTEX_POINT('',#53098);
#11326=VERTEX_POINT('',#53100);
#11327=VERTEX_POINT('',#53104);
#11328=VERTEX_POINT('',#53106);
#11329=VERTEX_POINT('',#53110);
#11330=VERTEX_POINT('',#53112);
#11331=VERTEX_POINT('',#53116);
#11332=VERTEX_POINT('',#53118);
#11333=VERTEX_POINT('',#53122);
#11334=VERTEX_POINT('',#53124);
#11335=VERTEX_POINT('',#53128);
#11336=VERTEX_POINT('',#53130);
#11337=VERTEX_POINT('',#53134);
#11338=VERTEX_POINT('',#53136);
#11339=VERTEX_POINT('',#53140);
#11340=VERTEX_POINT('',#53142);
#11341=VERTEX_POINT('',#53146);
#11342=VERTEX_POINT('',#53148);
#11343=VERTEX_POINT('',#53152);
#11344=VERTEX_POINT('',#53154);
#11345=VERTEX_POINT('',#53158);
#11346=VERTEX_POINT('',#53160);
#11347=VERTEX_POINT('',#53164);
#11348=VERTEX_POINT('',#53166);
#11349=VERTEX_POINT('',#53170);
#11350=VERTEX_POINT('',#53172);
#11351=VERTEX_POINT('',#53176);
#11352=VERTEX_POINT('',#53178);
#11353=VERTEX_POINT('',#53182);
#11354=VERTEX_POINT('',#53184);
#11355=VERTEX_POINT('',#53188);
#11356=VERTEX_POINT('',#53190);
#11357=VERTEX_POINT('',#53194);
#11358=VERTEX_POINT('',#53196);
#11359=VERTEX_POINT('',#53200);
#11360=VERTEX_POINT('',#53202);
#11361=VERTEX_POINT('',#53206);
#11362=VERTEX_POINT('',#53208);
#11363=VERTEX_POINT('',#53212);
#11364=VERTEX_POINT('',#53214);
#11365=VERTEX_POINT('',#53218);
#11366=VERTEX_POINT('',#53220);
#11367=VERTEX_POINT('',#53224);
#11368=VERTEX_POINT('',#53226);
#11369=VERTEX_POINT('',#53230);
#11370=VERTEX_POINT('',#53232);
#11371=VERTEX_POINT('',#53236);
#11372=VERTEX_POINT('',#53238);
#11373=VERTEX_POINT('',#53242);
#11374=VERTEX_POINT('',#53244);
#11375=VERTEX_POINT('',#53248);
#11376=VERTEX_POINT('',#53250);
#11377=VERTEX_POINT('',#53254);
#11378=VERTEX_POINT('',#53256);
#11379=VERTEX_POINT('',#53260);
#11380=VERTEX_POINT('',#53262);
#11381=VERTEX_POINT('',#53266);
#11382=VERTEX_POINT('',#53268);
#11383=VERTEX_POINT('',#53272);
#11384=VERTEX_POINT('',#53274);
#11385=VERTEX_POINT('',#53278);
#11386=VERTEX_POINT('',#53280);
#11387=VERTEX_POINT('',#53284);
#11388=VERTEX_POINT('',#53286);
#11389=VERTEX_POINT('',#53290);
#11390=VERTEX_POINT('',#53292);
#11391=VERTEX_POINT('',#53296);
#11392=VERTEX_POINT('',#53298);
#11393=VERTEX_POINT('',#53302);
#11394=VERTEX_POINT('',#53304);
#11395=VERTEX_POINT('',#53308);
#11396=VERTEX_POINT('',#53310);
#11397=VERTEX_POINT('',#53314);
#11398=VERTEX_POINT('',#53316);
#11399=VERTEX_POINT('',#53320);
#11400=VERTEX_POINT('',#53322);
#11401=VERTEX_POINT('',#53326);
#11402=VERTEX_POINT('',#53328);
#11403=VERTEX_POINT('',#53332);
#11404=VERTEX_POINT('',#53334);
#11405=VERTEX_POINT('',#53338);
#11406=VERTEX_POINT('',#53340);
#11407=VERTEX_POINT('',#53344);
#11408=VERTEX_POINT('',#53346);
#11409=VERTEX_POINT('',#53350);
#11410=VERTEX_POINT('',#53351);
#11411=VERTEX_POINT('',#53353);
#11412=VERTEX_POINT('',#53355);
#11413=VERTEX_POINT('',#53357);
#11414=VERTEX_POINT('',#53359);
#11415=VERTEX_POINT('',#53361);
#11416=VERTEX_POINT('',#53363);
#11417=VERTEX_POINT('',#53367);
#11418=VERTEX_POINT('',#53368);
#11419=VERTEX_POINT('',#53370);
#11420=VERTEX_POINT('',#53372);
#11421=VERTEX_POINT('',#53376);
#11422=VERTEX_POINT('',#53377);
#11423=VERTEX_POINT('',#53379);
#11424=VERTEX_POINT('',#53381);
#11425=VERTEX_POINT('',#53385);
#11426=VERTEX_POINT('',#53386);
#11427=VERTEX_POINT('',#53388);
#11428=VERTEX_POINT('',#53390);
#11429=VERTEX_POINT('',#53397);
#11430=VERTEX_POINT('',#53399);
#11431=VERTEX_POINT('',#53406);
#11432=VERTEX_POINT('',#53408);
#11433=VERTEX_POINT('',#53412);
#11434=VERTEX_POINT('',#53413);
#11435=VERTEX_POINT('',#53415);
#11436=VERTEX_POINT('',#53417);
#11437=VERTEX_POINT('',#53419);
#11438=VERTEX_POINT('',#53421);
#11439=VERTEX_POINT('',#53423);
#11440=VERTEX_POINT('',#53425);
#14081=EDGE_CURVE('',#11289,#11290,#6035,.T.);
#14082=EDGE_CURVE('',#11291,#11289,#6036,.T.);
#14083=EDGE_CURVE('',#11291,#11292,#6037,.T.);
#14084=EDGE_CURVE('',#11292,#11290,#6038,.T.);
#14085=EDGE_CURVE('',#11293,#11289,#6039,.T.);
#14086=EDGE_CURVE('',#11294,#11293,#6040,.T.);
#14087=EDGE_CURVE('',#11294,#11291,#6041,.T.);
#14088=EDGE_CURVE('',#11295,#11293,#6042,.T.);
#14089=EDGE_CURVE('',#11296,#11295,#6043,.T.);
#14090=EDGE_CURVE('',#11296,#11294,#6044,.T.);
#14091=EDGE_CURVE('',#11295,#11297,#6045,.T.);
#14092=EDGE_CURVE('',#11298,#11297,#6046,.T.);
#14093=EDGE_CURVE('',#11296,#11298,#6047,.T.);
#14094=EDGE_CURVE('',#11297,#11290,#6048,.T.);
#14095=EDGE_CURVE('',#11298,#11292,#6049,.T.);
#14096=EDGE_CURVE('',#11299,#11300,#6050,.T.);
#14097=EDGE_CURVE('',#11301,#11300,#6051,.T.);
#14098=EDGE_CURVE('',#11302,#11301,#6052,.T.);
#14099=EDGE_CURVE('',#11302,#11299,#6053,.T.);
#14100=EDGE_CURVE('',#11303,#11299,#6054,.T.);
#14101=EDGE_CURVE('',#11304,#11302,#6055,.T.);
#14102=EDGE_CURVE('',#11304,#11303,#6056,.T.);
#14103=EDGE_CURVE('',#11305,#11303,#6057,.T.);
#14104=EDGE_CURVE('',#11306,#11304,#6058,.T.);
#14105=EDGE_CURVE('',#11306,#11305,#6059,.T.);
#14106=EDGE_CURVE('',#11305,#11307,#6060,.T.);
#14107=EDGE_CURVE('',#11306,#11308,#6061,.T.);
#14108=EDGE_CURVE('',#11308,#11307,#6062,.T.);
#14109=EDGE_CURVE('',#11307,#11300,#6063,.T.);
#14110=EDGE_CURVE('',#11308,#11301,#6064,.T.);
#14111=EDGE_CURVE('',#11309,#11310,#9708,.T.);
#14112=EDGE_CURVE('',#11310,#11311,#6065,.T.);
#14113=EDGE_CURVE('',#11311,#11312,#9709,.T.);
#14114=EDGE_CURVE('',#11309,#11312,#6066,.T.);
#14115=EDGE_CURVE('',#11313,#11313,#9710,.T.);
#14116=EDGE_CURVE('',#11313,#11314,#6067,.T.);
#14117=EDGE_CURVE('',#11314,#11314,#9711,.T.);
#14118=EDGE_CURVE('',#11315,#11315,#9712,.T.);
#14119=EDGE_CURVE('',#11315,#11316,#6068,.T.);
#14120=EDGE_CURVE('',#11316,#11316,#9713,.T.);
#14121=EDGE_CURVE('',#11317,#11317,#9714,.T.);
#14122=EDGE_CURVE('',#11317,#11318,#6069,.T.);
#14123=EDGE_CURVE('',#11318,#11318,#9715,.T.);
#14124=EDGE_CURVE('',#11319,#11319,#9716,.T.);
#14125=EDGE_CURVE('',#11319,#11320,#6070,.T.);
#14126=EDGE_CURVE('',#11320,#11320,#9717,.T.);
#14127=EDGE_CURVE('',#11321,#11321,#9718,.T.);
#14128=EDGE_CURVE('',#11321,#11322,#6071,.T.);
#14129=EDGE_CURVE('',#11322,#11322,#9719,.T.);
#14130=EDGE_CURVE('',#11323,#11323,#9720,.T.);
#14131=EDGE_CURVE('',#11323,#11324,#6072,.T.);
#14132=EDGE_CURVE('',#11324,#11324,#9721,.T.);
#14133=EDGE_CURVE('',#11325,#11325,#9722,.T.);
#14134=EDGE_CURVE('',#11325,#11326,#6073,.T.);
#14135=EDGE_CURVE('',#11326,#11326,#9723,.T.);
#14136=EDGE_CURVE('',#11327,#11327,#9724,.T.);
#14137=EDGE_CURVE('',#11327,#11328,#6074,.T.);
#14138=EDGE_CURVE('',#11328,#11328,#9725,.T.);
#14139=EDGE_CURVE('',#11329,#11329,#9726,.T.);
#14140=EDGE_CURVE('',#11329,#11330,#6075,.T.);
#14141=EDGE_CURVE('',#11330,#11330,#9727,.T.);
#14142=EDGE_CURVE('',#11331,#11331,#9728,.T.);
#14143=EDGE_CURVE('',#11331,#11332,#6076,.T.);
#14144=EDGE_CURVE('',#11332,#11332,#9729,.T.);
#14145=EDGE_CURVE('',#11333,#11333,#9730,.T.);
#14146=EDGE_CURVE('',#11333,#11334,#6077,.T.);
#14147=EDGE_CURVE('',#11334,#11334,#9731,.T.);
#14148=EDGE_CURVE('',#11335,#11335,#9732,.T.);
#14149=EDGE_CURVE('',#11335,#11336,#6078,.T.);
#14150=EDGE_CURVE('',#11336,#11336,#9733,.T.);
#14151=EDGE_CURVE('',#11337,#11337,#9734,.T.);
#14152=EDGE_CURVE('',#11337,#11338,#6079,.T.);
#14153=EDGE_CURVE('',#11338,#11338,#9735,.T.);
#14154=EDGE_CURVE('',#11339,#11339,#9736,.T.);
#14155=EDGE_CURVE('',#11339,#11340,#6080,.T.);
#14156=EDGE_CURVE('',#11340,#11340,#9737,.T.);
#14157=EDGE_CURVE('',#11341,#11341,#9738,.T.);
#14158=EDGE_CURVE('',#11341,#11342,#6081,.T.);
#14159=EDGE_CURVE('',#11342,#11342,#9739,.T.);
#14160=EDGE_CURVE('',#11343,#11343,#9740,.T.);
#14161=EDGE_CURVE('',#11343,#11344,#6082,.T.);
#14162=EDGE_CURVE('',#11344,#11344,#9741,.T.);
#14163=EDGE_CURVE('',#11345,#11345,#9742,.T.);
#14164=EDGE_CURVE('',#11345,#11346,#6083,.T.);
#14165=EDGE_CURVE('',#11346,#11346,#9743,.T.);
#14166=EDGE_CURVE('',#11347,#11347,#9744,.T.);
#14167=EDGE_CURVE('',#11347,#11348,#6084,.T.);
#14168=EDGE_CURVE('',#11348,#11348,#9745,.T.);
#14169=EDGE_CURVE('',#11349,#11349,#9746,.T.);
#14170=EDGE_CURVE('',#11349,#11350,#6085,.T.);
#14171=EDGE_CURVE('',#11350,#11350,#9747,.T.);
#14172=EDGE_CURVE('',#11351,#11351,#9748,.T.);
#14173=EDGE_CURVE('',#11351,#11352,#6086,.T.);
#14174=EDGE_CURVE('',#11352,#11352,#9749,.T.);
#14175=EDGE_CURVE('',#11353,#11353,#9750,.T.);
#14176=EDGE_CURVE('',#11353,#11354,#6087,.T.);
#14177=EDGE_CURVE('',#11354,#11354,#9751,.T.);
#14178=EDGE_CURVE('',#11355,#11355,#9752,.T.);
#14179=EDGE_CURVE('',#11355,#11356,#6088,.T.);
#14180=EDGE_CURVE('',#11356,#11356,#9753,.T.);
#14181=EDGE_CURVE('',#11357,#11357,#9754,.T.);
#14182=EDGE_CURVE('',#11357,#11358,#6089,.T.);
#14183=EDGE_CURVE('',#11358,#11358,#9755,.T.);
#14184=EDGE_CURVE('',#11359,#11359,#9756,.T.);
#14185=EDGE_CURVE('',#11359,#11360,#6090,.T.);
#14186=EDGE_CURVE('',#11360,#11360,#9757,.T.);
#14187=EDGE_CURVE('',#11361,#11361,#9758,.T.);
#14188=EDGE_CURVE('',#11361,#11362,#6091,.T.);
#14189=EDGE_CURVE('',#11362,#11362,#9759,.T.);
#14190=EDGE_CURVE('',#11363,#11363,#9760,.T.);
#14191=EDGE_CURVE('',#11363,#11364,#6092,.T.);
#14192=EDGE_CURVE('',#11364,#11364,#9761,.T.);
#14193=EDGE_CURVE('',#11365,#11365,#9762,.T.);
#14194=EDGE_CURVE('',#11365,#11366,#6093,.T.);
#14195=EDGE_CURVE('',#11366,#11366,#9763,.T.);
#14196=EDGE_CURVE('',#11367,#11367,#9764,.T.);
#14197=EDGE_CURVE('',#11367,#11368,#6094,.T.);
#14198=EDGE_CURVE('',#11368,#11368,#9765,.T.);
#14199=EDGE_CURVE('',#11369,#11369,#9766,.T.);
#14200=EDGE_CURVE('',#11369,#11370,#6095,.T.);
#14201=EDGE_CURVE('',#11370,#11370,#9767,.T.);
#14202=EDGE_CURVE('',#11371,#11371,#9768,.T.);
#14203=EDGE_CURVE('',#11371,#11372,#6096,.T.);
#14204=EDGE_CURVE('',#11372,#11372,#9769,.T.);
#14205=EDGE_CURVE('',#11373,#11373,#9770,.T.);
#14206=EDGE_CURVE('',#11373,#11374,#6097,.T.);
#14207=EDGE_CURVE('',#11374,#11374,#9771,.T.);
#14208=EDGE_CURVE('',#11375,#11375,#9772,.T.);
#14209=EDGE_CURVE('',#11375,#11376,#6098,.T.);
#14210=EDGE_CURVE('',#11376,#11376,#9773,.T.);
#14211=EDGE_CURVE('',#11377,#11377,#9774,.T.);
#14212=EDGE_CURVE('',#11377,#11378,#6099,.T.);
#14213=EDGE_CURVE('',#11378,#11378,#9775,.T.);
#14214=EDGE_CURVE('',#11379,#11379,#9776,.T.);
#14215=EDGE_CURVE('',#11379,#11380,#6100,.T.);
#14216=EDGE_CURVE('',#11380,#11380,#9777,.T.);
#14217=EDGE_CURVE('',#11381,#11381,#9778,.T.);
#14218=EDGE_CURVE('',#11381,#11382,#6101,.T.);
#14219=EDGE_CURVE('',#11382,#11382,#9779,.T.);
#14220=EDGE_CURVE('',#11383,#11383,#9780,.T.);
#14221=EDGE_CURVE('',#11383,#11384,#6102,.T.);
#14222=EDGE_CURVE('',#11384,#11384,#9781,.T.);
#14223=EDGE_CURVE('',#11385,#11385,#9782,.T.);
#14224=EDGE_CURVE('',#11385,#11386,#6103,.T.);
#14225=EDGE_CURVE('',#11386,#11386,#9783,.T.);
#14226=EDGE_CURVE('',#11387,#11387,#9784,.T.);
#14227=EDGE_CURVE('',#11387,#11388,#6104,.T.);
#14228=EDGE_CURVE('',#11388,#11388,#9785,.T.);
#14229=EDGE_CURVE('',#11389,#11389,#9786,.T.);
#14230=EDGE_CURVE('',#11389,#11390,#6105,.T.);
#14231=EDGE_CURVE('',#11390,#11390,#9787,.T.);
#14232=EDGE_CURVE('',#11391,#11391,#9788,.T.);
#14233=EDGE_CURVE('',#11391,#11392,#6106,.T.);
#14234=EDGE_CURVE('',#11392,#11392,#9789,.T.);
#14235=EDGE_CURVE('',#11393,#11393,#9790,.T.);
#14236=EDGE_CURVE('',#11393,#11394,#6107,.T.);
#14237=EDGE_CURVE('',#11394,#11394,#9791,.T.);
#14238=EDGE_CURVE('',#11395,#11395,#9792,.T.);
#14239=EDGE_CURVE('',#11395,#11396,#6108,.T.);
#14240=EDGE_CURVE('',#11396,#11396,#9793,.T.);
#14241=EDGE_CURVE('',#11397,#11397,#9794,.T.);
#14242=EDGE_CURVE('',#11397,#11398,#6109,.T.);
#14243=EDGE_CURVE('',#11398,#11398,#9795,.T.);
#14244=EDGE_CURVE('',#11399,#11399,#9796,.T.);
#14245=EDGE_CURVE('',#11399,#11400,#6110,.T.);
#14246=EDGE_CURVE('',#11400,#11400,#9797,.T.);
#14247=EDGE_CURVE('',#11401,#11401,#9798,.T.);
#14248=EDGE_CURVE('',#11401,#11402,#6111,.T.);
#14249=EDGE_CURVE('',#11402,#11402,#9799,.T.);
#14250=EDGE_CURVE('',#11403,#11403,#9800,.T.);
#14251=EDGE_CURVE('',#11403,#11404,#6112,.T.);
#14252=EDGE_CURVE('',#11404,#11404,#9801,.T.);
#14253=EDGE_CURVE('',#11405,#11405,#9802,.T.);
#14254=EDGE_CURVE('',#11405,#11406,#6113,.T.);
#14255=EDGE_CURVE('',#11406,#11406,#9803,.T.);
#14256=EDGE_CURVE('',#11407,#11407,#9804,.T.);
#14257=EDGE_CURVE('',#11407,#11408,#6114,.T.);
#14258=EDGE_CURVE('',#11408,#11408,#9805,.T.);
#14259=EDGE_CURVE('',#11409,#11410,#6115,.T.);
#14260=EDGE_CURVE('',#11409,#11411,#6116,.T.);
#14261=EDGE_CURVE('',#11412,#11411,#6117,.T.);
#14262=EDGE_CURVE('',#11412,#11413,#6118,.T.);
#14263=EDGE_CURVE('',#11414,#11413,#6119,.T.);
#14264=EDGE_CURVE('',#11414,#11415,#6120,.T.);
#14265=EDGE_CURVE('',#11416,#11415,#6121,.T.);
#14266=EDGE_CURVE('',#11416,#11410,#6122,.T.);
#14267=EDGE_CURVE('',#11417,#11418,#6123,.T.);
#14268=EDGE_CURVE('',#11418,#11419,#6124,.T.);
#14269=EDGE_CURVE('',#11420,#11419,#6125,.T.);
#14270=EDGE_CURVE('',#11420,#11417,#6126,.T.);
#14271=EDGE_CURVE('',#11421,#11422,#6127,.T.);
#14272=EDGE_CURVE('',#11421,#11423,#6128,.T.);
#14273=EDGE_CURVE('',#11423,#11424,#6129,.T.);
#14274=EDGE_CURVE('',#11424,#11422,#6130,.T.);
#14275=EDGE_CURVE('',#11425,#11426,#6131,.T.);
#14276=EDGE_CURVE('',#11426,#11427,#6132,.T.);
#14277=EDGE_CURVE('',#11428,#11427,#6133,.T.);
#14278=EDGE_CURVE('',#11425,#11428,#6134,.T.);
#14279=EDGE_CURVE('',#11419,#11421,#6135,.T.);
#14280=EDGE_CURVE('',#11422,#11426,#6136,.T.);
#14281=EDGE_CURVE('',#11425,#11420,#6137,.T.);
#14282=EDGE_CURVE('',#11310,#11429,#6138,.T.);
#14283=EDGE_CURVE('',#11430,#11309,#6139,.T.);
#14284=EDGE_CURVE('',#11429,#11430,#9806,.T.);
#14285=EDGE_CURVE('',#11423,#11418,#6140,.T.);
#14286=EDGE_CURVE('',#11428,#11417,#6141,.T.);
#14287=EDGE_CURVE('',#11427,#11424,#6142,.T.);
#14288=EDGE_CURVE('',#11431,#11311,#6143,.T.);
#14289=EDGE_CURVE('',#11432,#11431,#9807,.T.);
#14290=EDGE_CURVE('',#11312,#11432,#6144,.T.);
#14291=EDGE_CURVE('',#11433,#11434,#6145,.T.);
#14292=EDGE_CURVE('',#11434,#11435,#6146,.T.);
#14293=EDGE_CURVE('',#11435,#11436,#6147,.T.);
#14294=EDGE_CURVE('',#11436,#11437,#6148,.T.);
#14295=EDGE_CURVE('',#11437,#11438,#6149,.T.);
#14296=EDGE_CURVE('',#11438,#11439,#6150,.T.);
#14297=EDGE_CURVE('',#11439,#11440,#6151,.T.);
#14298=EDGE_CURVE('',#11440,#11433,#6152,.T.);
#14299=EDGE_CURVE('',#11435,#11409,#6153,.T.);
#14300=EDGE_CURVE('',#11410,#11436,#6154,.T.);
#14301=EDGE_CURVE('',#11415,#11438,#6155,.T.);
#14302=EDGE_CURVE('',#11437,#11416,#6156,.T.);
#14303=EDGE_CURVE('',#11413,#11440,#6157,.T.);
#14304=EDGE_CURVE('',#11439,#11414,#6158,.T.);
#14305=EDGE_CURVE('',#11411,#11434,#6159,.T.);
#14306=EDGE_CURVE('',#11433,#11412,#6160,.T.);
#14307=EDGE_CURVE('',#11429,#11431,#6161,.T.);
#14308=EDGE_CURVE('',#11430,#11432,#6162,.T.);
#19072=ORIENTED_EDGE('',*,*,#14081,.F.);
#19073=ORIENTED_EDGE('',*,*,#14082,.F.);
#19074=ORIENTED_EDGE('',*,*,#14083,.T.);
#19075=ORIENTED_EDGE('',*,*,#14084,.T.);
#19076=ORIENTED_EDGE('',*,*,#14085,.F.);
#19077=ORIENTED_EDGE('',*,*,#14086,.F.);
#19078=ORIENTED_EDGE('',*,*,#14087,.T.);
#19079=ORIENTED_EDGE('',*,*,#14082,.T.);
#19080=ORIENTED_EDGE('',*,*,#14088,.F.);
#19081=ORIENTED_EDGE('',*,*,#14089,.F.);
#19082=ORIENTED_EDGE('',*,*,#14090,.T.);
#19083=ORIENTED_EDGE('',*,*,#14086,.T.);
#19084=ORIENTED_EDGE('',*,*,#14091,.T.);
#19085=ORIENTED_EDGE('',*,*,#14092,.F.);
#19086=ORIENTED_EDGE('',*,*,#14093,.F.);
#19087=ORIENTED_EDGE('',*,*,#14089,.T.);
#19088=ORIENTED_EDGE('',*,*,#14094,.T.);
#19089=ORIENTED_EDGE('',*,*,#14084,.F.);
#19090=ORIENTED_EDGE('',*,*,#14095,.F.);
#19091=ORIENTED_EDGE('',*,*,#14092,.T.);
#19092=ORIENTED_EDGE('',*,*,#14083,.F.);
#19093=ORIENTED_EDGE('',*,*,#14087,.F.);
#19094=ORIENTED_EDGE('',*,*,#14090,.F.);
#19095=ORIENTED_EDGE('',*,*,#14093,.T.);
#19096=ORIENTED_EDGE('',*,*,#14095,.T.);
#19097=ORIENTED_EDGE('',*,*,#14081,.T.);
#19098=ORIENTED_EDGE('',*,*,#14094,.F.);
#19099=ORIENTED_EDGE('',*,*,#14091,.F.);
#19100=ORIENTED_EDGE('',*,*,#14088,.T.);
#19101=ORIENTED_EDGE('',*,*,#14085,.T.);
#19102=ORIENTED_EDGE('',*,*,#14096,.T.);
#19103=ORIENTED_EDGE('',*,*,#14097,.F.);
#19104=ORIENTED_EDGE('',*,*,#14098,.F.);
#19105=ORIENTED_EDGE('',*,*,#14099,.T.);
#19106=ORIENTED_EDGE('',*,*,#14100,.T.);
#19107=ORIENTED_EDGE('',*,*,#14099,.F.);
#19108=ORIENTED_EDGE('',*,*,#14101,.F.);
#19109=ORIENTED_EDGE('',*,*,#14102,.T.);
#19110=ORIENTED_EDGE('',*,*,#14103,.T.);
#19111=ORIENTED_EDGE('',*,*,#14102,.F.);
#19112=ORIENTED_EDGE('',*,*,#14104,.F.);
#19113=ORIENTED_EDGE('',*,*,#14105,.T.);
#19114=ORIENTED_EDGE('',*,*,#14106,.F.);
#19115=ORIENTED_EDGE('',*,*,#14105,.F.);
#19116=ORIENTED_EDGE('',*,*,#14107,.T.);
#19117=ORIENTED_EDGE('',*,*,#14108,.T.);
#19118=ORIENTED_EDGE('',*,*,#14109,.F.);
#19119=ORIENTED_EDGE('',*,*,#14108,.F.);
#19120=ORIENTED_EDGE('',*,*,#14110,.T.);
#19121=ORIENTED_EDGE('',*,*,#14097,.T.);
#19122=ORIENTED_EDGE('',*,*,#14098,.T.);
#19123=ORIENTED_EDGE('',*,*,#14110,.F.);
#19124=ORIENTED_EDGE('',*,*,#14107,.F.);
#19125=ORIENTED_EDGE('',*,*,#14104,.T.);
#19126=ORIENTED_EDGE('',*,*,#14101,.T.);
#19127=ORIENTED_EDGE('',*,*,#14096,.F.);
#19128=ORIENTED_EDGE('',*,*,#14100,.F.);
#19129=ORIENTED_EDGE('',*,*,#14103,.F.);
#19130=ORIENTED_EDGE('',*,*,#14106,.T.);
#19131=ORIENTED_EDGE('',*,*,#14109,.T.);
#19132=ORIENTED_EDGE('',*,*,#14111,.T.);
#19133=ORIENTED_EDGE('',*,*,#14112,.T.);
#19134=ORIENTED_EDGE('',*,*,#14113,.T.);
#19135=ORIENTED_EDGE('',*,*,#14114,.F.);
#19136=ORIENTED_EDGE('',*,*,#14115,.T.);
#19137=ORIENTED_EDGE('',*,*,#14116,.T.);
#19138=ORIENTED_EDGE('',*,*,#14117,.T.);
#19139=ORIENTED_EDGE('',*,*,#14116,.F.);
#19140=ORIENTED_EDGE('',*,*,#14118,.T.);
#19141=ORIENTED_EDGE('',*,*,#14119,.T.);
#19142=ORIENTED_EDGE('',*,*,#14120,.T.);
#19143=ORIENTED_EDGE('',*,*,#14119,.F.);
#19144=ORIENTED_EDGE('',*,*,#14121,.T.);
#19145=ORIENTED_EDGE('',*,*,#14122,.T.);
#19146=ORIENTED_EDGE('',*,*,#14123,.T.);
#19147=ORIENTED_EDGE('',*,*,#14122,.F.);
#19148=ORIENTED_EDGE('',*,*,#14124,.T.);
#19149=ORIENTED_EDGE('',*,*,#14125,.T.);
#19150=ORIENTED_EDGE('',*,*,#14126,.T.);
#19151=ORIENTED_EDGE('',*,*,#14125,.F.);
#19152=ORIENTED_EDGE('',*,*,#14127,.T.);
#19153=ORIENTED_EDGE('',*,*,#14128,.T.);
#19154=ORIENTED_EDGE('',*,*,#14129,.T.);
#19155=ORIENTED_EDGE('',*,*,#14128,.F.);
#19156=ORIENTED_EDGE('',*,*,#14130,.T.);
#19157=ORIENTED_EDGE('',*,*,#14131,.T.);
#19158=ORIENTED_EDGE('',*,*,#14132,.T.);
#19159=ORIENTED_EDGE('',*,*,#14131,.F.);
#19160=ORIENTED_EDGE('',*,*,#14133,.T.);
#19161=ORIENTED_EDGE('',*,*,#14134,.T.);
#19162=ORIENTED_EDGE('',*,*,#14135,.T.);
#19163=ORIENTED_EDGE('',*,*,#14134,.F.);
#19164=ORIENTED_EDGE('',*,*,#14136,.T.);
#19165=ORIENTED_EDGE('',*,*,#14137,.T.);
#19166=ORIENTED_EDGE('',*,*,#14138,.T.);
#19167=ORIENTED_EDGE('',*,*,#14137,.F.);
#19168=ORIENTED_EDGE('',*,*,#14139,.T.);
#19169=ORIENTED_EDGE('',*,*,#14140,.T.);
#19170=ORIENTED_EDGE('',*,*,#14141,.T.);
#19171=ORIENTED_EDGE('',*,*,#14140,.F.);
#19172=ORIENTED_EDGE('',*,*,#14142,.F.);
#19173=ORIENTED_EDGE('',*,*,#14143,.T.);
#19174=ORIENTED_EDGE('',*,*,#14144,.T.);
#19175=ORIENTED_EDGE('',*,*,#14143,.F.);
#19176=ORIENTED_EDGE('',*,*,#14145,.T.);
#19177=ORIENTED_EDGE('',*,*,#14146,.T.);
#19178=ORIENTED_EDGE('',*,*,#14147,.T.);
#19179=ORIENTED_EDGE('',*,*,#14146,.F.);
#19180=ORIENTED_EDGE('',*,*,#14148,.T.);
#19181=ORIENTED_EDGE('',*,*,#14149,.T.);
#19182=ORIENTED_EDGE('',*,*,#14150,.T.);
#19183=ORIENTED_EDGE('',*,*,#14149,.F.);
#19184=ORIENTED_EDGE('',*,*,#14151,.T.);
#19185=ORIENTED_EDGE('',*,*,#14152,.T.);
#19186=ORIENTED_EDGE('',*,*,#14153,.T.);
#19187=ORIENTED_EDGE('',*,*,#14152,.F.);
#19188=ORIENTED_EDGE('',*,*,#14154,.T.);
#19189=ORIENTED_EDGE('',*,*,#14155,.T.);
#19190=ORIENTED_EDGE('',*,*,#14156,.T.);
#19191=ORIENTED_EDGE('',*,*,#14155,.F.);
#19192=ORIENTED_EDGE('',*,*,#14157,.T.);
#19193=ORIENTED_EDGE('',*,*,#14158,.T.);
#19194=ORIENTED_EDGE('',*,*,#14159,.T.);
#19195=ORIENTED_EDGE('',*,*,#14158,.F.);
#19196=ORIENTED_EDGE('',*,*,#14160,.T.);
#19197=ORIENTED_EDGE('',*,*,#14161,.T.);
#19198=ORIENTED_EDGE('',*,*,#14162,.T.);
#19199=ORIENTED_EDGE('',*,*,#14161,.F.);
#19200=ORIENTED_EDGE('',*,*,#14163,.F.);
#19201=ORIENTED_EDGE('',*,*,#14164,.T.);
#19202=ORIENTED_EDGE('',*,*,#14165,.T.);
#19203=ORIENTED_EDGE('',*,*,#14164,.F.);
#19204=ORIENTED_EDGE('',*,*,#14166,.F.);
#19205=ORIENTED_EDGE('',*,*,#14167,.T.);
#19206=ORIENTED_EDGE('',*,*,#14168,.T.);
#19207=ORIENTED_EDGE('',*,*,#14167,.F.);
#19208=ORIENTED_EDGE('',*,*,#14169,.F.);
#19209=ORIENTED_EDGE('',*,*,#14170,.T.);
#19210=ORIENTED_EDGE('',*,*,#14171,.T.);
#19211=ORIENTED_EDGE('',*,*,#14170,.F.);
#19212=ORIENTED_EDGE('',*,*,#14172,.F.);
#19213=ORIENTED_EDGE('',*,*,#14173,.T.);
#19214=ORIENTED_EDGE('',*,*,#14174,.T.);
#19215=ORIENTED_EDGE('',*,*,#14173,.F.);
#19216=ORIENTED_EDGE('',*,*,#14175,.F.);
#19217=ORIENTED_EDGE('',*,*,#14176,.T.);
#19218=ORIENTED_EDGE('',*,*,#14177,.T.);
#19219=ORIENTED_EDGE('',*,*,#14176,.F.);
#19220=ORIENTED_EDGE('',*,*,#14178,.F.);
#19221=ORIENTED_EDGE('',*,*,#14179,.T.);
#19222=ORIENTED_EDGE('',*,*,#14180,.T.);
#19223=ORIENTED_EDGE('',*,*,#14179,.F.);
#19224=ORIENTED_EDGE('',*,*,#14181,.F.);
#19225=ORIENTED_EDGE('',*,*,#14182,.T.);
#19226=ORIENTED_EDGE('',*,*,#14183,.T.);
#19227=ORIENTED_EDGE('',*,*,#14182,.F.);
#19228=ORIENTED_EDGE('',*,*,#14184,.F.);
#19229=ORIENTED_EDGE('',*,*,#14185,.T.);
#19230=ORIENTED_EDGE('',*,*,#14186,.T.);
#19231=ORIENTED_EDGE('',*,*,#14185,.F.);
#19232=ORIENTED_EDGE('',*,*,#14187,.F.);
#19233=ORIENTED_EDGE('',*,*,#14188,.T.);
#19234=ORIENTED_EDGE('',*,*,#14189,.T.);
#19235=ORIENTED_EDGE('',*,*,#14188,.F.);
#19236=ORIENTED_EDGE('',*,*,#14190,.F.);
#19237=ORIENTED_EDGE('',*,*,#14191,.T.);
#19238=ORIENTED_EDGE('',*,*,#14192,.T.);
#19239=ORIENTED_EDGE('',*,*,#14191,.F.);
#19240=ORIENTED_EDGE('',*,*,#14193,.F.);
#19241=ORIENTED_EDGE('',*,*,#14194,.T.);
#19242=ORIENTED_EDGE('',*,*,#14195,.T.);
#19243=ORIENTED_EDGE('',*,*,#14194,.F.);
#19244=ORIENTED_EDGE('',*,*,#14196,.F.);
#19245=ORIENTED_EDGE('',*,*,#14197,.T.);
#19246=ORIENTED_EDGE('',*,*,#14198,.T.);
#19247=ORIENTED_EDGE('',*,*,#14197,.F.);
#19248=ORIENTED_EDGE('',*,*,#14199,.F.);
#19249=ORIENTED_EDGE('',*,*,#14200,.T.);
#19250=ORIENTED_EDGE('',*,*,#14201,.T.);
#19251=ORIENTED_EDGE('',*,*,#14200,.F.);
#19252=ORIENTED_EDGE('',*,*,#14202,.F.);
#19253=ORIENTED_EDGE('',*,*,#14203,.T.);
#19254=ORIENTED_EDGE('',*,*,#14204,.T.);
#19255=ORIENTED_EDGE('',*,*,#14203,.F.);
#19256=ORIENTED_EDGE('',*,*,#14205,.F.);
#19257=ORIENTED_EDGE('',*,*,#14206,.T.);
#19258=ORIENTED_EDGE('',*,*,#14207,.T.);
#19259=ORIENTED_EDGE('',*,*,#14206,.F.);
#19260=ORIENTED_EDGE('',*,*,#14208,.F.);
#19261=ORIENTED_EDGE('',*,*,#14209,.T.);
#19262=ORIENTED_EDGE('',*,*,#14210,.T.);
#19263=ORIENTED_EDGE('',*,*,#14209,.F.);
#19264=ORIENTED_EDGE('',*,*,#14211,.F.);
#19265=ORIENTED_EDGE('',*,*,#14212,.T.);
#19266=ORIENTED_EDGE('',*,*,#14213,.T.);
#19267=ORIENTED_EDGE('',*,*,#14212,.F.);
#19268=ORIENTED_EDGE('',*,*,#14214,.F.);
#19269=ORIENTED_EDGE('',*,*,#14215,.T.);
#19270=ORIENTED_EDGE('',*,*,#14216,.T.);
#19271=ORIENTED_EDGE('',*,*,#14215,.F.);
#19272=ORIENTED_EDGE('',*,*,#14217,.F.);
#19273=ORIENTED_EDGE('',*,*,#14218,.T.);
#19274=ORIENTED_EDGE('',*,*,#14219,.T.);
#19275=ORIENTED_EDGE('',*,*,#14218,.F.);
#19276=ORIENTED_EDGE('',*,*,#14220,.F.);
#19277=ORIENTED_EDGE('',*,*,#14221,.T.);
#19278=ORIENTED_EDGE('',*,*,#14222,.T.);
#19279=ORIENTED_EDGE('',*,*,#14221,.F.);
#19280=ORIENTED_EDGE('',*,*,#14223,.F.);
#19281=ORIENTED_EDGE('',*,*,#14224,.T.);
#19282=ORIENTED_EDGE('',*,*,#14225,.T.);
#19283=ORIENTED_EDGE('',*,*,#14224,.F.);
#19284=ORIENTED_EDGE('',*,*,#14226,.F.);
#19285=ORIENTED_EDGE('',*,*,#14227,.T.);
#19286=ORIENTED_EDGE('',*,*,#14228,.T.);
#19287=ORIENTED_EDGE('',*,*,#14227,.F.);
#19288=ORIENTED_EDGE('',*,*,#14229,.F.);
#19289=ORIENTED_EDGE('',*,*,#14230,.T.);
#19290=ORIENTED_EDGE('',*,*,#14231,.T.);
#19291=ORIENTED_EDGE('',*,*,#14230,.F.);
#19292=ORIENTED_EDGE('',*,*,#14232,.F.);
#19293=ORIENTED_EDGE('',*,*,#14233,.T.);
#19294=ORIENTED_EDGE('',*,*,#14234,.T.);
#19295=ORIENTED_EDGE('',*,*,#14233,.F.);
#19296=ORIENTED_EDGE('',*,*,#14235,.F.);
#19297=ORIENTED_EDGE('',*,*,#14236,.T.);
#19298=ORIENTED_EDGE('',*,*,#14237,.T.);
#19299=ORIENTED_EDGE('',*,*,#14236,.F.);
#19300=ORIENTED_EDGE('',*,*,#14238,.F.);
#19301=ORIENTED_EDGE('',*,*,#14239,.T.);
#19302=ORIENTED_EDGE('',*,*,#14240,.T.);
#19303=ORIENTED_EDGE('',*,*,#14239,.F.);
#19304=ORIENTED_EDGE('',*,*,#14241,.F.);
#19305=ORIENTED_EDGE('',*,*,#14242,.T.);
#19306=ORIENTED_EDGE('',*,*,#14243,.T.);
#19307=ORIENTED_EDGE('',*,*,#14242,.F.);
#19308=ORIENTED_EDGE('',*,*,#14244,.F.);
#19309=ORIENTED_EDGE('',*,*,#14245,.T.);
#19310=ORIENTED_EDGE('',*,*,#14246,.T.);
#19311=ORIENTED_EDGE('',*,*,#14245,.F.);
#19312=ORIENTED_EDGE('',*,*,#14247,.F.);
#19313=ORIENTED_EDGE('',*,*,#14248,.T.);
#19314=ORIENTED_EDGE('',*,*,#14249,.T.);
#19315=ORIENTED_EDGE('',*,*,#14248,.F.);
#19316=ORIENTED_EDGE('',*,*,#14250,.F.);
#19317=ORIENTED_EDGE('',*,*,#14251,.T.);
#19318=ORIENTED_EDGE('',*,*,#14252,.T.);
#19319=ORIENTED_EDGE('',*,*,#14251,.F.);
#19320=ORIENTED_EDGE('',*,*,#14253,.F.);
#19321=ORIENTED_EDGE('',*,*,#14254,.T.);
#19322=ORIENTED_EDGE('',*,*,#14255,.T.);
#19323=ORIENTED_EDGE('',*,*,#14254,.F.);
#19324=ORIENTED_EDGE('',*,*,#14256,.F.);
#19325=ORIENTED_EDGE('',*,*,#14257,.T.);
#19326=ORIENTED_EDGE('',*,*,#14258,.T.);
#19327=ORIENTED_EDGE('',*,*,#14257,.F.);
#19328=ORIENTED_EDGE('',*,*,#14259,.F.);
#19329=ORIENTED_EDGE('',*,*,#14260,.T.);
#19330=ORIENTED_EDGE('',*,*,#14261,.F.);
#19331=ORIENTED_EDGE('',*,*,#14262,.T.);
#19332=ORIENTED_EDGE('',*,*,#14263,.F.);
#19333=ORIENTED_EDGE('',*,*,#14264,.T.);
#19334=ORIENTED_EDGE('',*,*,#14265,.F.);
#19335=ORIENTED_EDGE('',*,*,#14266,.T.);
#19336=ORIENTED_EDGE('',*,*,#14256,.T.);
#19337=ORIENTED_EDGE('',*,*,#14250,.T.);
#19338=ORIENTED_EDGE('',*,*,#14244,.T.);
#19339=ORIENTED_EDGE('',*,*,#14238,.T.);
#19340=ORIENTED_EDGE('',*,*,#14232,.T.);
#19341=ORIENTED_EDGE('',*,*,#14226,.T.);
#19342=ORIENTED_EDGE('',*,*,#14220,.T.);
#19343=ORIENTED_EDGE('',*,*,#14166,.T.);
#19344=ORIENTED_EDGE('',*,*,#14147,.F.);
#19345=ORIENTED_EDGE('',*,*,#14150,.F.);
#19346=ORIENTED_EDGE('',*,*,#14153,.F.);
#19347=ORIENTED_EDGE('',*,*,#14156,.F.);
#19348=ORIENTED_EDGE('',*,*,#14159,.F.);
#19349=ORIENTED_EDGE('',*,*,#14162,.F.);
#19350=ORIENTED_EDGE('',*,*,#14172,.T.);
#19351=ORIENTED_EDGE('',*,*,#14178,.T.);
#19352=ORIENTED_EDGE('',*,*,#14184,.T.);
#19353=ORIENTED_EDGE('',*,*,#14190,.T.);
#19354=ORIENTED_EDGE('',*,*,#14196,.T.);
#19355=ORIENTED_EDGE('',*,*,#14202,.T.);
#19356=ORIENTED_EDGE('',*,*,#14208,.T.);
#19357=ORIENTED_EDGE('',*,*,#14214,.T.);
#19358=ORIENTED_EDGE('',*,*,#14267,.T.);
#19359=ORIENTED_EDGE('',*,*,#14268,.T.);
#19360=ORIENTED_EDGE('',*,*,#14269,.F.);
#19361=ORIENTED_EDGE('',*,*,#14270,.T.);
#19362=ORIENTED_EDGE('',*,*,#14271,.F.);
#19363=ORIENTED_EDGE('',*,*,#14272,.T.);
#19364=ORIENTED_EDGE('',*,*,#14273,.T.);
#19365=ORIENTED_EDGE('',*,*,#14274,.T.);
#19366=ORIENTED_EDGE('',*,*,#14275,.T.);
#19367=ORIENTED_EDGE('',*,*,#14276,.T.);
#19368=ORIENTED_EDGE('',*,*,#14277,.F.);
#19369=ORIENTED_EDGE('',*,*,#14278,.F.);
#19370=ORIENTED_EDGE('',*,*,#14269,.T.);
#19371=ORIENTED_EDGE('',*,*,#14279,.T.);
#19372=ORIENTED_EDGE('',*,*,#14271,.T.);
#19373=ORIENTED_EDGE('',*,*,#14280,.T.);
#19374=ORIENTED_EDGE('',*,*,#14275,.F.);
#19375=ORIENTED_EDGE('',*,*,#14281,.T.);
#19376=ORIENTED_EDGE('',*,*,#14117,.F.);
#19377=ORIENTED_EDGE('',*,*,#14120,.F.);
#19378=ORIENTED_EDGE('',*,*,#14123,.F.);
#19379=ORIENTED_EDGE('',*,*,#14126,.F.);
#19380=ORIENTED_EDGE('',*,*,#14282,.F.);
#19381=ORIENTED_EDGE('',*,*,#14111,.F.);
#19382=ORIENTED_EDGE('',*,*,#14283,.F.);
#19383=ORIENTED_EDGE('',*,*,#14284,.F.);
#19384=ORIENTED_EDGE('',*,*,#14129,.F.);
#19385=ORIENTED_EDGE('',*,*,#14132,.F.);
#19386=ORIENTED_EDGE('',*,*,#14135,.F.);
#19387=ORIENTED_EDGE('',*,*,#14138,.F.);
#19388=ORIENTED_EDGE('',*,*,#14144,.F.);
#19389=ORIENTED_EDGE('',*,*,#14273,.F.);
#19390=ORIENTED_EDGE('',*,*,#14285,.T.);
#19391=ORIENTED_EDGE('',*,*,#14267,.F.);
#19392=ORIENTED_EDGE('',*,*,#14286,.F.);
#19393=ORIENTED_EDGE('',*,*,#14277,.T.);
#19394=ORIENTED_EDGE('',*,*,#14287,.T.);
#19395=ORIENTED_EDGE('',*,*,#14113,.F.);
#19396=ORIENTED_EDGE('',*,*,#14288,.F.);
#19397=ORIENTED_EDGE('',*,*,#14289,.F.);
#19398=ORIENTED_EDGE('',*,*,#14290,.F.);
#19399=ORIENTED_EDGE('',*,*,#14115,.F.);
#19400=ORIENTED_EDGE('',*,*,#14118,.F.);
#19401=ORIENTED_EDGE('',*,*,#14121,.F.);
#19402=ORIENTED_EDGE('',*,*,#14124,.F.);
#19403=ORIENTED_EDGE('',*,*,#14127,.F.);
#19404=ORIENTED_EDGE('',*,*,#14130,.F.);
#19405=ORIENTED_EDGE('',*,*,#14133,.F.);
#19406=ORIENTED_EDGE('',*,*,#14136,.F.);
#19407=ORIENTED_EDGE('',*,*,#14139,.F.);
#19408=ORIENTED_EDGE('',*,*,#14291,.T.);
#19409=ORIENTED_EDGE('',*,*,#14292,.T.);
#19410=ORIENTED_EDGE('',*,*,#14293,.T.);
#19411=ORIENTED_EDGE('',*,*,#14294,.T.);
#19412=ORIENTED_EDGE('',*,*,#14295,.T.);
#19413=ORIENTED_EDGE('',*,*,#14296,.T.);
#19414=ORIENTED_EDGE('',*,*,#14297,.T.);
#19415=ORIENTED_EDGE('',*,*,#14298,.T.);
#19416=ORIENTED_EDGE('',*,*,#14281,.F.);
#19417=ORIENTED_EDGE('',*,*,#14278,.T.);
#19418=ORIENTED_EDGE('',*,*,#14286,.T.);
#19419=ORIENTED_EDGE('',*,*,#14270,.F.);
#19420=ORIENTED_EDGE('',*,*,#14145,.F.);
#19421=ORIENTED_EDGE('',*,*,#14148,.F.);
#19422=ORIENTED_EDGE('',*,*,#14151,.F.);
#19423=ORIENTED_EDGE('',*,*,#14154,.F.);
#19424=ORIENTED_EDGE('',*,*,#14157,.F.);
#19425=ORIENTED_EDGE('',*,*,#14160,.F.);
#19426=ORIENTED_EDGE('',*,*,#14165,.F.);
#19427=ORIENTED_EDGE('',*,*,#14171,.F.);
#19428=ORIENTED_EDGE('',*,*,#14177,.F.);
#19429=ORIENTED_EDGE('',*,*,#14183,.F.);
#19430=ORIENTED_EDGE('',*,*,#14189,.F.);
#19431=ORIENTED_EDGE('',*,*,#14195,.F.);
#19432=ORIENTED_EDGE('',*,*,#14201,.F.);
#19433=ORIENTED_EDGE('',*,*,#14207,.F.);
#19434=ORIENTED_EDGE('',*,*,#14213,.F.);
#19435=ORIENTED_EDGE('',*,*,#14219,.F.);
#19436=ORIENTED_EDGE('',*,*,#14225,.F.);
#19437=ORIENTED_EDGE('',*,*,#14231,.F.);
#19438=ORIENTED_EDGE('',*,*,#14237,.F.);
#19439=ORIENTED_EDGE('',*,*,#14243,.F.);
#19440=ORIENTED_EDGE('',*,*,#14249,.F.);
#19441=ORIENTED_EDGE('',*,*,#14255,.F.);
#19442=ORIENTED_EDGE('',*,*,#14293,.F.);
#19443=ORIENTED_EDGE('',*,*,#14299,.T.);
#19444=ORIENTED_EDGE('',*,*,#14259,.T.);
#19445=ORIENTED_EDGE('',*,*,#14300,.T.);
#19446=ORIENTED_EDGE('',*,*,#14265,.T.);
#19447=ORIENTED_EDGE('',*,*,#14301,.T.);
#19448=ORIENTED_EDGE('',*,*,#14295,.F.);
#19449=ORIENTED_EDGE('',*,*,#14302,.T.);
#19450=ORIENTED_EDGE('',*,*,#14263,.T.);
#19451=ORIENTED_EDGE('',*,*,#14303,.T.);
#19452=ORIENTED_EDGE('',*,*,#14297,.F.);
#19453=ORIENTED_EDGE('',*,*,#14304,.T.);
#19454=ORIENTED_EDGE('',*,*,#14261,.T.);
#19455=ORIENTED_EDGE('',*,*,#14305,.T.);
#19456=ORIENTED_EDGE('',*,*,#14291,.F.);
#19457=ORIENTED_EDGE('',*,*,#14306,.T.);
#19458=ORIENTED_EDGE('',*,*,#14253,.T.);
#19459=ORIENTED_EDGE('',*,*,#14258,.F.);
#19460=ORIENTED_EDGE('',*,*,#14247,.T.);
#19461=ORIENTED_EDGE('',*,*,#14252,.F.);
#19462=ORIENTED_EDGE('',*,*,#14241,.T.);
#19463=ORIENTED_EDGE('',*,*,#14246,.F.);
#19464=ORIENTED_EDGE('',*,*,#14235,.T.);
#19465=ORIENTED_EDGE('',*,*,#14240,.F.);
#19466=ORIENTED_EDGE('',*,*,#14229,.T.);
#19467=ORIENTED_EDGE('',*,*,#14234,.F.);
#19468=ORIENTED_EDGE('',*,*,#14223,.T.);
#19469=ORIENTED_EDGE('',*,*,#14228,.F.);
#19470=ORIENTED_EDGE('',*,*,#14217,.T.);
#19471=ORIENTED_EDGE('',*,*,#14222,.F.);
#19472=ORIENTED_EDGE('',*,*,#14211,.T.);
#19473=ORIENTED_EDGE('',*,*,#14216,.F.);
#19474=ORIENTED_EDGE('',*,*,#14205,.T.);
#19475=ORIENTED_EDGE('',*,*,#14210,.F.);
#19476=ORIENTED_EDGE('',*,*,#14199,.T.);
#19477=ORIENTED_EDGE('',*,*,#14204,.F.);
#19478=ORIENTED_EDGE('',*,*,#14193,.T.);
#19479=ORIENTED_EDGE('',*,*,#14198,.F.);
#19480=ORIENTED_EDGE('',*,*,#14187,.T.);
#19481=ORIENTED_EDGE('',*,*,#14192,.F.);
#19482=ORIENTED_EDGE('',*,*,#14181,.T.);
#19483=ORIENTED_EDGE('',*,*,#14186,.F.);
#19484=ORIENTED_EDGE('',*,*,#14175,.T.);
#19485=ORIENTED_EDGE('',*,*,#14180,.F.);
#19486=ORIENTED_EDGE('',*,*,#14169,.T.);
#19487=ORIENTED_EDGE('',*,*,#14174,.F.);
#19488=ORIENTED_EDGE('',*,*,#14163,.T.);
#19489=ORIENTED_EDGE('',*,*,#14168,.F.);
#19490=ORIENTED_EDGE('',*,*,#14142,.T.);
#19491=ORIENTED_EDGE('',*,*,#14141,.F.);
#19492=ORIENTED_EDGE('',*,*,#14279,.F.);
#19493=ORIENTED_EDGE('',*,*,#14268,.F.);
#19494=ORIENTED_EDGE('',*,*,#14285,.F.);
#19495=ORIENTED_EDGE('',*,*,#14272,.F.);
#19496=ORIENTED_EDGE('',*,*,#14280,.F.);
#19497=ORIENTED_EDGE('',*,*,#14274,.F.);
#19498=ORIENTED_EDGE('',*,*,#14287,.F.);
#19499=ORIENTED_EDGE('',*,*,#14276,.F.);
#19500=ORIENTED_EDGE('',*,*,#14282,.T.);
#19501=ORIENTED_EDGE('',*,*,#14307,.T.);
#19502=ORIENTED_EDGE('',*,*,#14288,.T.);
#19503=ORIENTED_EDGE('',*,*,#14112,.F.);
#19504=ORIENTED_EDGE('',*,*,#14283,.T.);
#19505=ORIENTED_EDGE('',*,*,#14114,.T.);
#19506=ORIENTED_EDGE('',*,*,#14290,.T.);
#19507=ORIENTED_EDGE('',*,*,#14308,.F.);
#19508=ORIENTED_EDGE('',*,*,#14284,.T.);
#19509=ORIENTED_EDGE('',*,*,#14308,.T.);
#19510=ORIENTED_EDGE('',*,*,#14289,.T.);
#19511=ORIENTED_EDGE('',*,*,#14307,.F.);
#19512=ORIENTED_EDGE('',*,*,#14292,.F.);
#19513=ORIENTED_EDGE('',*,*,#14305,.F.);
#19514=ORIENTED_EDGE('',*,*,#14260,.F.);
#19515=ORIENTED_EDGE('',*,*,#14299,.F.);
#19516=ORIENTED_EDGE('',*,*,#14298,.F.);
#19517=ORIENTED_EDGE('',*,*,#14303,.F.);
#19518=ORIENTED_EDGE('',*,*,#14262,.F.);
#19519=ORIENTED_EDGE('',*,*,#14306,.F.);
#19520=ORIENTED_EDGE('',*,*,#14296,.F.);
#19521=ORIENTED_EDGE('',*,*,#14301,.F.);
#19522=ORIENTED_EDGE('',*,*,#14264,.F.);
#19523=ORIENTED_EDGE('',*,*,#14304,.F.);
#19524=ORIENTED_EDGE('',*,*,#14294,.F.);
#19525=ORIENTED_EDGE('',*,*,#14300,.F.);
#19526=ORIENTED_EDGE('',*,*,#14266,.F.);
#19527=ORIENTED_EDGE('',*,*,#14302,.F.);
#22908=CYLINDRICAL_SURFACE('',#26083,55.);
#22909=CYLINDRICAL_SURFACE('',#26086,3.39999999999999);
#22910=CYLINDRICAL_SURFACE('',#26089,3.4);
#22911=CYLINDRICAL_SURFACE('',#26092,3.4);
#22912=CYLINDRICAL_SURFACE('',#26095,3.39999999999999);
#22913=CYLINDRICAL_SURFACE('',#26098,4.24999999999998);
#22914=CYLINDRICAL_SURFACE('',#26101,4.24999999999998);
#22915=CYLINDRICAL_SURFACE('',#26104,4.24999999999998);
#22916=CYLINDRICAL_SURFACE('',#26107,4.24999999999998);
#22917=CYLINDRICAL_SURFACE('',#26110,45.);
#22918=CYLINDRICAL_SURFACE('',#26113,65.);
#22919=CYLINDRICAL_SURFACE('',#26116,2.99999999999999);
#22920=CYLINDRICAL_SURFACE('',#26119,2.99999999999999);
#22921=CYLINDRICAL_SURFACE('',#26122,2.5);
#22922=CYLINDRICAL_SURFACE('',#26125,2.5);
#22923=CYLINDRICAL_SURFACE('',#26128,2.5);
#22924=CYLINDRICAL_SURFACE('',#26131,2.5);
#22925=CYLINDRICAL_SURFACE('',#26134,5.50000000000001);
#22926=CYLINDRICAL_SURFACE('',#26137,3.30000000000004);
#22927=CYLINDRICAL_SURFACE('',#26140,5.50000000000001);
#22928=CYLINDRICAL_SURFACE('',#26143,3.30000000000004);
#22929=CYLINDRICAL_SURFACE('',#26146,5.50000000000001);
#22930=CYLINDRICAL_SURFACE('',#26149,3.30000000000004);
#22931=CYLINDRICAL_SURFACE('',#26152,5.50000000000001);
#22932=CYLINDRICAL_SURFACE('',#26155,3.30000000000004);
#22933=CYLINDRICAL_SURFACE('',#26158,5.50000000000001);
#22934=CYLINDRICAL_SURFACE('',#26161,3.30000000000004);
#22935=CYLINDRICAL_SURFACE('',#26164,5.50000000000001);
#22936=CYLINDRICAL_SURFACE('',#26167,3.30000000000004);
#22937=CYLINDRICAL_SURFACE('',#26170,5.49999999999999);
#22938=CYLINDRICAL_SURFACE('',#26173,3.30000000000004);
#22939=CYLINDRICAL_SURFACE('',#26176,5.50000000000001);
#22940=CYLINDRICAL_SURFACE('',#26179,3.30000000000004);
#22941=CYLINDRICAL_SURFACE('',#26182,5.50000000000001);
#22942=CYLINDRICAL_SURFACE('',#26185,3.30000000000004);
#22943=CYLINDRICAL_SURFACE('',#26188,5.50000000000001);
#22944=CYLINDRICAL_SURFACE('',#26191,3.30000000000004);
#22945=CYLINDRICAL_SURFACE('',#26194,5.50000000000001);
#22946=CYLINDRICAL_SURFACE('',#26197,3.30000000000004);
#22947=CYLINDRICAL_SURFACE('',#26200,5.50000000000001);
#22948=CYLINDRICAL_SURFACE('',#26203,3.30000000000004);
#22949=CYLINDRICAL_SURFACE('',#26206,5.50000000000001);
#22950=CYLINDRICAL_SURFACE('',#26209,3.30000000000004);
#22951=CYLINDRICAL_SURFACE('',#26212,5.50000000000001);
#22952=CYLINDRICAL_SURFACE('',#26215,3.30000000000004);
#22953=CYLINDRICAL_SURFACE('',#26218,5.49999999999999);
#22954=CYLINDRICAL_SURFACE('',#26221,3.30000000000004);
#22955=CYLINDRICAL_SURFACE('',#26224,5.50000000000001);
#22956=CYLINDRICAL_SURFACE('',#26227,3.30000000000004);
#22957=CYLINDRICAL_SURFACE('',#26264,55.);
#23818=ADVANCED_FACE('',(#2826),#1680,.T.);
#23819=ADVANCED_FACE('',(#2827),#1681,.T.);
#23820=ADVANCED_FACE('',(#2828),#1682,.T.);
#23821=ADVANCED_FACE('',(#2829),#1683,.F.);
#23822=ADVANCED_FACE('',(#2830),#1684,.F.);
#23823=ADVANCED_FACE('',(#2831),#1685,.T.);
#23824=ADVANCED_FACE('',(#2832),#1686,.F.);
#23825=ADVANCED_FACE('',(#2833),#1687,.T.);
#23826=ADVANCED_FACE('',(#2834),#1688,.T.);
#23827=ADVANCED_FACE('',(#2835),#1689,.T.);
#23828=ADVANCED_FACE('',(#2836),#1690,.F.);
#23829=ADVANCED_FACE('',(#2837),#1691,.F.);
#23830=ADVANCED_FACE('',(#2838),#1692,.T.);
#23831=ADVANCED_FACE('',(#2839),#1693,.F.);
#23832=ADVANCED_FACE('',(#2840),#22908,.F.);
#23833=ADVANCED_FACE('',(#2841),#22909,.F.);
#23834=ADVANCED_FACE('',(#2842),#22910,.F.);
#23835=ADVANCED_FACE('',(#2843),#22911,.F.);
#23836=ADVANCED_FACE('',(#2844),#22912,.F.);
#23837=ADVANCED_FACE('',(#2845),#22913,.F.);
#23838=ADVANCED_FACE('',(#2846),#22914,.F.);
#23839=ADVANCED_FACE('',(#2847),#22915,.F.);
#23840=ADVANCED_FACE('',(#2848),#22916,.F.);
#23841=ADVANCED_FACE('',(#2849),#22917,.F.);
#23842=ADVANCED_FACE('',(#2850),#22918,.F.);
#23843=ADVANCED_FACE('',(#2851),#22919,.F.);
#23844=ADVANCED_FACE('',(#2852),#22920,.F.);
#23845=ADVANCED_FACE('',(#2853),#22921,.F.);
#23846=ADVANCED_FACE('',(#2854),#22922,.F.);
#23847=ADVANCED_FACE('',(#2855),#22923,.F.);
#23848=ADVANCED_FACE('',(#2856),#22924,.F.);
#23849=ADVANCED_FACE('',(#2857),#22925,.F.);
#23850=ADVANCED_FACE('',(#2858),#22926,.F.);
#23851=ADVANCED_FACE('',(#2859),#22927,.F.);
#23852=ADVANCED_FACE('',(#2860),#22928,.F.);
#23853=ADVANCED_FACE('',(#2861),#22929,.F.);
#23854=ADVANCED_FACE('',(#2862),#22930,.F.);
#23855=ADVANCED_FACE('',(#2863),#22931,.F.);
#23856=ADVANCED_FACE('',(#2864),#22932,.F.);
#23857=ADVANCED_FACE('',(#2865),#22933,.F.);
#23858=ADVANCED_FACE('',(#2866),#22934,.F.);
#23859=ADVANCED_FACE('',(#2867),#22935,.F.);
#23860=ADVANCED_FACE('',(#2868),#22936,.F.);
#23861=ADVANCED_FACE('',(#2869),#22937,.F.);
#23862=ADVANCED_FACE('',(#2870),#22938,.F.);
#23863=ADVANCED_FACE('',(#2871),#22939,.F.);
#23864=ADVANCED_FACE('',(#2872),#22940,.F.);
#23865=ADVANCED_FACE('',(#2873),#22941,.F.);
#23866=ADVANCED_FACE('',(#2874),#22942,.F.);
#23867=ADVANCED_FACE('',(#2875),#22943,.F.);
#23868=ADVANCED_FACE('',(#2876),#22944,.F.);
#23869=ADVANCED_FACE('',(#2877),#22945,.F.);
#23870=ADVANCED_FACE('',(#2878),#22946,.F.);
#23871=ADVANCED_FACE('',(#2879),#22947,.F.);
#23872=ADVANCED_FACE('',(#2880),#22948,.F.);
#23873=ADVANCED_FACE('',(#2881),#22949,.F.);
#23874=ADVANCED_FACE('',(#2882),#22950,.F.);
#23875=ADVANCED_FACE('',(#2883),#22951,.F.);
#23876=ADVANCED_FACE('',(#2884),#22952,.F.);
#23877=ADVANCED_FACE('',(#2885),#22953,.F.);
#23878=ADVANCED_FACE('',(#2886),#22954,.F.);
#23879=ADVANCED_FACE('',(#2887),#22955,.F.);
#23880=ADVANCED_FACE('',(#2888),#22956,.F.);
#23881=ADVANCED_FACE('',(#2889,#1195,#1196,#1197,#1198,#1199,#1200,#1201,
#1202,#1203,#1204,#1205,#1206,#1207,#1208,#1209,#1210,#1211,#1212,#1213,
#1214,#1215,#1216),#1694,.T.);
#23882=ADVANCED_FACE('',(#2890),#1695,.F.);
#23883=ADVANCED_FACE('',(#2891),#1696,.F.);
#23884=ADVANCED_FACE('',(#2892),#1697,.T.);
#23885=ADVANCED_FACE('',(#2893,#1217,#1218,#1219,#1220,#1221,#1222,#1223,
#1224,#1225,#1226),#1698,.F.);
#23886=ADVANCED_FACE('',(#2894,#1227,#1228,#1229,#1230,#1231,#1232,#1233,
#1234,#1235,#1236),#1699,.T.);
#23887=ADVANCED_FACE('',(#2895,#1237,#1238,#1239,#1240,#1241,#1242,#1243,
#1244,#1245,#1246,#1247,#1248,#1249,#1250,#1251,#1252,#1253,#1254,#1255,
#1256,#1257,#1258,#1259),#1700,.T.);
#23888=ADVANCED_FACE('',(#2896),#1701,.F.);
#23889=ADVANCED_FACE('',(#2897),#1702,.F.);
#23890=ADVANCED_FACE('',(#2898),#1703,.F.);
#23891=ADVANCED_FACE('',(#2899),#1704,.F.);
#23892=ADVANCED_FACE('',(#2900,#1260),#1705,.F.);
#23893=ADVANCED_FACE('',(#2901,#1261),#1706,.F.);
#23894=ADVANCED_FACE('',(#2902,#1262),#1707,.F.);
#23895=ADVANCED_FACE('',(#2903,#1263),#1708,.F.);
#23896=ADVANCED_FACE('',(#2904,#1264),#1709,.F.);
#23897=ADVANCED_FACE('',(#2905,#1265),#1710,.F.);
#23898=ADVANCED_FACE('',(#2906,#1266),#1711,.F.);
#23899=ADVANCED_FACE('',(#2907,#1267),#1712,.F.);
#23900=ADVANCED_FACE('',(#2908,#1268),#1713,.F.);
#23901=ADVANCED_FACE('',(#2909,#1269),#1714,.F.);
#23902=ADVANCED_FACE('',(#2910,#1270),#1715,.F.);
#23903=ADVANCED_FACE('',(#2911,#1271),#1716,.F.);
#23904=ADVANCED_FACE('',(#2912,#1272),#1717,.F.);
#23905=ADVANCED_FACE('',(#2913,#1273),#1718,.F.);
#23906=ADVANCED_FACE('',(#2914,#1274),#1719,.F.);
#23907=ADVANCED_FACE('',(#2915,#1275),#1720,.F.);
#23908=ADVANCED_FACE('',(#2916,#1276),#1721,.T.);
#23909=ADVANCED_FACE('',(#2917),#1722,.F.);
#23910=ADVANCED_FACE('',(#2918),#1723,.T.);
#23911=ADVANCED_FACE('',(#2919),#1724,.F.);
#23912=ADVANCED_FACE('',(#2920),#1725,.F.);
#23913=ADVANCED_FACE('',(#2921),#22957,.F.);
#23914=ADVANCED_FACE('',(#2922),#1726,.F.);
#23915=ADVANCED_FACE('',(#2923),#1727,.F.);
#23916=ADVANCED_FACE('',(#2924),#1728,.F.);
#23917=ADVANCED_FACE('',(#2925),#1729,.F.);
#24547=CLOSED_SHELL('',(#23818,#23819,#23820,#23821,#23822,#23823,#23824));
#24548=CLOSED_SHELL('',(#23825,#23826,#23827,#23828,#23829,#23830,#23831));
#24549=CLOSED_SHELL('',(#23832,#23833,#23834,#23835,#23836,#23837,#23838,
#23839,#23840,#23841,#23842,#23843,#23844,#23845,#23846,#23847,#23848,#23849,
#23850,#23851,#23852,#23853,#23854,#23855,#23856,#23857,#23858,#23859,#23860,
#23861,#23862,#23863,#23864,#23865,#23866,#23867,#23868,#23869,#23870,#23871,
#23872,#23873,#23874,#23875,#23876,#23877,#23878,#23879,#23880,#23881,#23882,
#23883,#23884,#23885,#23886,#23887,#23888,#23889,#23890,#23891,#23892,#23893,
#23894,#23895,#23896,#23897,#23898,#23899,#23900,#23901,#23902,#23903,#23904,
#23905,#23906,#23907,#23908,#23909,#23910,#23911,#23912,#23913,#23914,#23915,
#23916,#23917));
#26068=AXIS2_PLACEMENT_3D('',#52987,#30631,#30632);
#26069=AXIS2_PLACEMENT_3D('',#52988,#30633,#30634);
#26070=AXIS2_PLACEMENT_3D('',#52997,#30639,#30640);
#26071=AXIS2_PLACEMENT_3D('',#53003,#30644,#30645);
#26072=AXIS2_PLACEMENT_3D('',#53009,#30649,#30650);
#26073=AXIS2_PLACEMENT_3D('',#53015,#30654,#30655);
#26074=AXIS2_PLACEMENT_3D('',#53018,#30658,#30659);
#26075=AXIS2_PLACEMENT_3D('',#53019,#30660,#30661);
#26076=AXIS2_PLACEMENT_3D('',#53020,#30662,#30663);
#26077=AXIS2_PLACEMENT_3D('',#53029,#30668,#30669);
#26078=AXIS2_PLACEMENT_3D('',#53035,#30673,#30674);
#26079=AXIS2_PLACEMENT_3D('',#53041,#30678,#30679);
#26080=AXIS2_PLACEMENT_3D('',#53047,#30683,#30684);
#26081=AXIS2_PLACEMENT_3D('',#53050,#30687,#30688);
#26082=AXIS2_PLACEMENT_3D('',#53051,#30689,#30690);
#26083=AXIS2_PLACEMENT_3D('',#53052,#30691,#30692);
#26084=AXIS2_PLACEMENT_3D('',#53055,#30693,#30694);
#26085=AXIS2_PLACEMENT_3D('',#53059,#30696,#30697);
#26086=AXIS2_PLACEMENT_3D('',#53061,#30699,#30700);
#26087=AXIS2_PLACEMENT_3D('',#53063,#30701,#30702);
#26088=AXIS2_PLACEMENT_3D('',#53066,#30704,#30705);
#26089=AXIS2_PLACEMENT_3D('',#53067,#30706,#30707);
#26090=AXIS2_PLACEMENT_3D('',#53069,#30708,#30709);
#26091=AXIS2_PLACEMENT_3D('',#53072,#30711,#30712);
#26092=AXIS2_PLACEMENT_3D('',#53073,#30713,#30714);
#26093=AXIS2_PLACEMENT_3D('',#53075,#30715,#30716);
#26094=AXIS2_PLACEMENT_3D('',#53078,#30718,#30719);
#26095=AXIS2_PLACEMENT_3D('',#53079,#30720,#30721);
#26096=AXIS2_PLACEMENT_3D('',#53081,#30722,#30723);
#26097=AXIS2_PLACEMENT_3D('',#53084,#30725,#30726);
#26098=AXIS2_PLACEMENT_3D('',#53085,#30727,#30728);
#26099=AXIS2_PLACEMENT_3D('',#53087,#30729,#30730);
#26100=AXIS2_PLACEMENT_3D('',#53090,#30732,#30733);
#26101=AXIS2_PLACEMENT_3D('',#53091,#30734,#30735);
#26102=AXIS2_PLACEMENT_3D('',#53093,#30736,#30737);
#26103=AXIS2_PLACEMENT_3D('',#53096,#30739,#30740);
#26104=AXIS2_PLACEMENT_3D('',#53097,#30741,#30742);
#26105=AXIS2_PLACEMENT_3D('',#53099,#30743,#30744);
#26106=AXIS2_PLACEMENT_3D('',#53102,#30746,#30747);
#26107=AXIS2_PLACEMENT_3D('',#53103,#30748,#30749);
#26108=AXIS2_PLACEMENT_3D('',#53105,#30750,#30751);
#26109=AXIS2_PLACEMENT_3D('',#53108,#30753,#30754);
#26110=AXIS2_PLACEMENT_3D('',#53109,#30755,#30756);
#26111=AXIS2_PLACEMENT_3D('',#53111,#30757,#30758);
#26112=AXIS2_PLACEMENT_3D('',#53114,#30760,#30761);
#26113=AXIS2_PLACEMENT_3D('',#53115,#30762,#30763);
#26114=AXIS2_PLACEMENT_3D('',#53117,#30764,#30765);
#26115=AXIS2_PLACEMENT_3D('',#53120,#30767,#30768);
#26116=AXIS2_PLACEMENT_3D('',#53121,#30769,#30770);
#26117=AXIS2_PLACEMENT_3D('',#53123,#30771,#30772);
#26118=AXIS2_PLACEMENT_3D('',#53126,#30774,#30775);
#26119=AXIS2_PLACEMENT_3D('',#53127,#30776,#30777);
#26120=AXIS2_PLACEMENT_3D('',#53129,#30778,#30779);
#26121=AXIS2_PLACEMENT_3D('',#53132,#30781,#30782);
#26122=AXIS2_PLACEMENT_3D('',#53133,#30783,#30784);
#26123=AXIS2_PLACEMENT_3D('',#53135,#30785,#30786);
#26124=AXIS2_PLACEMENT_3D('',#53138,#30788,#30789);
#26125=AXIS2_PLACEMENT_3D('',#53139,#30790,#30791);
#26126=AXIS2_PLACEMENT_3D('',#53141,#30792,#30793);
#26127=AXIS2_PLACEMENT_3D('',#53144,#30795,#30796);
#26128=AXIS2_PLACEMENT_3D('',#53145,#30797,#30798);
#26129=AXIS2_PLACEMENT_3D('',#53147,#30799,#30800);
#26130=AXIS2_PLACEMENT_3D('',#53150,#30802,#30803);
#26131=AXIS2_PLACEMENT_3D('',#53151,#30804,#30805);
#26132=AXIS2_PLACEMENT_3D('',#53153,#30806,#30807);
#26133=AXIS2_PLACEMENT_3D('',#53156,#30809,#30810);
#26134=AXIS2_PLACEMENT_3D('',#53157,#30811,#30812);
#26135=AXIS2_PLACEMENT_3D('',#53159,#30813,#30814);
#26136=AXIS2_PLACEMENT_3D('',#53162,#30816,#30817);
#26137=AXIS2_PLACEMENT_3D('',#53163,#30818,#30819);
#26138=AXIS2_PLACEMENT_3D('',#53165,#30820,#30821);
#26139=AXIS2_PLACEMENT_3D('',#53168,#30823,#30824);
#26140=AXIS2_PLACEMENT_3D('',#53169,#30825,#30826);
#26141=AXIS2_PLACEMENT_3D('',#53171,#30827,#30828);
#26142=AXIS2_PLACEMENT_3D('',#53174,#30830,#30831);
#26143=AXIS2_PLACEMENT_3D('',#53175,#30832,#30833);
#26144=AXIS2_PLACEMENT_3D('',#53177,#30834,#30835);
#26145=AXIS2_PLACEMENT_3D('',#53180,#30837,#30838);
#26146=AXIS2_PLACEMENT_3D('',#53181,#30839,#30840);
#26147=AXIS2_PLACEMENT_3D('',#53183,#30841,#30842);
#26148=AXIS2_PLACEMENT_3D('',#53186,#30844,#30845);
#26149=AXIS2_PLACEMENT_3D('',#53187,#30846,#30847);
#26150=AXIS2_PLACEMENT_3D('',#53189,#30848,#30849);
#26151=AXIS2_PLACEMENT_3D('',#53192,#30851,#30852);
#26152=AXIS2_PLACEMENT_3D('',#53193,#30853,#30854);
#26153=AXIS2_PLACEMENT_3D('',#53195,#30855,#30856);
#26154=AXIS2_PLACEMENT_3D('',#53198,#30858,#30859);
#26155=AXIS2_PLACEMENT_3D('',#53199,#30860,#30861);
#26156=AXIS2_PLACEMENT_3D('',#53201,#30862,#30863);
#26157=AXIS2_PLACEMENT_3D('',#53204,#30865,#30866);
#26158=AXIS2_PLACEMENT_3D('',#53205,#30867,#30868);
#26159=AXIS2_PLACEMENT_3D('',#53207,#30869,#30870);
#26160=AXIS2_PLACEMENT_3D('',#53210,#30872,#30873);
#26161=AXIS2_PLACEMENT_3D('',#53211,#30874,#30875);
#26162=AXIS2_PLACEMENT_3D('',#53213,#30876,#30877);
#26163=AXIS2_PLACEMENT_3D('',#53216,#30879,#30880);
#26164=AXIS2_PLACEMENT_3D('',#53217,#30881,#30882);
#26165=AXIS2_PLACEMENT_3D('',#53219,#30883,#30884);
#26166=AXIS2_PLACEMENT_3D('',#53222,#30886,#30887);
#26167=AXIS2_PLACEMENT_3D('',#53223,#30888,#30889);
#26168=AXIS2_PLACEMENT_3D('',#53225,#30890,#30891);
#26169=AXIS2_PLACEMENT_3D('',#53228,#30893,#30894);
#26170=AXIS2_PLACEMENT_3D('',#53229,#30895,#30896);
#26171=AXIS2_PLACEMENT_3D('',#53231,#30897,#30898);
#26172=AXIS2_PLACEMENT_3D('',#53234,#30900,#30901);
#26173=AXIS2_PLACEMENT_3D('',#53235,#30902,#30903);
#26174=AXIS2_PLACEMENT_3D('',#53237,#30904,#30905);
#26175=AXIS2_PLACEMENT_3D('',#53240,#30907,#30908);
#26176=AXIS2_PLACEMENT_3D('',#53241,#30909,#30910);
#26177=AXIS2_PLACEMENT_3D('',#53243,#30911,#30912);
#26178=AXIS2_PLACEMENT_3D('',#53246,#30914,#30915);
#26179=AXIS2_PLACEMENT_3D('',#53247,#30916,#30917);
#26180=AXIS2_PLACEMENT_3D('',#53249,#30918,#30919);
#26181=AXIS2_PLACEMENT_3D('',#53252,#30921,#30922);
#26182=AXIS2_PLACEMENT_3D('',#53253,#30923,#30924);
#26183=AXIS2_PLACEMENT_3D('',#53255,#30925,#30926);
#26184=AXIS2_PLACEMENT_3D('',#53258,#30928,#30929);
#26185=AXIS2_PLACEMENT_3D('',#53259,#30930,#30931);
#26186=AXIS2_PLACEMENT_3D('',#53261,#30932,#30933);
#26187=AXIS2_PLACEMENT_3D('',#53264,#30935,#30936);
#26188=AXIS2_PLACEMENT_3D('',#53265,#30937,#30938);
#26189=AXIS2_PLACEMENT_3D('',#53267,#30939,#30940);
#26190=AXIS2_PLACEMENT_3D('',#53270,#30942,#30943);
#26191=AXIS2_PLACEMENT_3D('',#53271,#30944,#30945);
#26192=AXIS2_PLACEMENT_3D('',#53273,#30946,#30947);
#26193=AXIS2_PLACEMENT_3D('',#53276,#30949,#30950);
#26194=AXIS2_PLACEMENT_3D('',#53277,#30951,#30952);
#26195=AXIS2_PLACEMENT_3D('',#53279,#30953,#30954);
#26196=AXIS2_PLACEMENT_3D('',#53282,#30956,#30957);
#26197=AXIS2_PLACEMENT_3D('',#53283,#30958,#30959);
#26198=AXIS2_PLACEMENT_3D('',#53285,#30960,#30961);
#26199=AXIS2_PLACEMENT_3D('',#53288,#30963,#30964);
#26200=AXIS2_PLACEMENT_3D('',#53289,#30965,#30966);
#26201=AXIS2_PLACEMENT_3D('',#53291,#30967,#30968);
#26202=AXIS2_PLACEMENT_3D('',#53294,#30970,#30971);
#26203=AXIS2_PLACEMENT_3D('',#53295,#30972,#30973);
#26204=AXIS2_PLACEMENT_3D('',#53297,#30974,#30975);
#26205=AXIS2_PLACEMENT_3D('',#53300,#30977,#30978);
#26206=AXIS2_PLACEMENT_3D('',#53301,#30979,#30980);
#26207=AXIS2_PLACEMENT_3D('',#53303,#30981,#30982);
#26208=AXIS2_PLACEMENT_3D('',#53306,#30984,#30985);
#26209=AXIS2_PLACEMENT_3D('',#53307,#30986,#30987);
#26210=AXIS2_PLACEMENT_3D('',#53309,#30988,#30989);
#26211=AXIS2_PLACEMENT_3D('',#53312,#30991,#30992);
#26212=AXIS2_PLACEMENT_3D('',#53313,#30993,#30994);
#26213=AXIS2_PLACEMENT_3D('',#53315,#30995,#30996);
#26214=AXIS2_PLACEMENT_3D('',#53318,#30998,#30999);
#26215=AXIS2_PLACEMENT_3D('',#53319,#31000,#31001);
#26216=AXIS2_PLACEMENT_3D('',#53321,#31002,#31003);
#26217=AXIS2_PLACEMENT_3D('',#53324,#31005,#31006);
#26218=AXIS2_PLACEMENT_3D('',#53325,#31007,#31008);
#26219=AXIS2_PLACEMENT_3D('',#53327,#31009,#31010);
#26220=AXIS2_PLACEMENT_3D('',#53330,#31012,#31013);
#26221=AXIS2_PLACEMENT_3D('',#53331,#31014,#31015);
#26222=AXIS2_PLACEMENT_3D('',#53333,#31016,#31017);
#26223=AXIS2_PLACEMENT_3D('',#53336,#31019,#31020);
#26224=AXIS2_PLACEMENT_3D('',#53337,#31021,#31022);
#26225=AXIS2_PLACEMENT_3D('',#53339,#31023,#31024);
#26226=AXIS2_PLACEMENT_3D('',#53342,#31026,#31027);
#26227=AXIS2_PLACEMENT_3D('',#53343,#31028,#31029);
#26228=AXIS2_PLACEMENT_3D('',#53345,#31030,#31031);
#26229=AXIS2_PLACEMENT_3D('',#53348,#31033,#31034);
#26230=AXIS2_PLACEMENT_3D('',#53349,#31035,#31036);
#26231=AXIS2_PLACEMENT_3D('',#53366,#31045,#31046);
#26232=AXIS2_PLACEMENT_3D('',#53375,#31051,#31052);
#26233=AXIS2_PLACEMENT_3D('',#53384,#31057,#31058);
#26234=AXIS2_PLACEMENT_3D('',#53393,#31063,#31064);
#26235=AXIS2_PLACEMENT_3D('',#53401,#31070,#31071);
#26236=AXIS2_PLACEMENT_3D('',#53402,#31072,#31073);
#26237=AXIS2_PLACEMENT_3D('',#53409,#31078,#31079);
#26238=AXIS2_PLACEMENT_3D('',#53411,#31081,#31082);
#26239=AXIS2_PLACEMENT_3D('',#53428,#31091,#31092);
#26240=AXIS2_PLACEMENT_3D('',#53431,#31095,#31096);
#26241=AXIS2_PLACEMENT_3D('',#53434,#31099,#31100);
#26242=AXIS2_PLACEMENT_3D('',#53437,#31103,#31104);
#26243=AXIS2_PLACEMENT_3D('',#53440,#31107,#31108);
#26244=AXIS2_PLACEMENT_3D('',#53441,#31109,#31110);
#26245=AXIS2_PLACEMENT_3D('',#53442,#31111,#31112);
#26246=AXIS2_PLACEMENT_3D('',#53443,#31113,#31114);
#26247=AXIS2_PLACEMENT_3D('',#53444,#31115,#31116);
#26248=AXIS2_PLACEMENT_3D('',#53445,#31117,#31118);
#26249=AXIS2_PLACEMENT_3D('',#53446,#31119,#31120);
#26250=AXIS2_PLACEMENT_3D('',#53447,#31121,#31122);
#26251=AXIS2_PLACEMENT_3D('',#53448,#31123,#31124);
#26252=AXIS2_PLACEMENT_3D('',#53449,#31125,#31126);
#26253=AXIS2_PLACEMENT_3D('',#53450,#31127,#31128);
#26254=AXIS2_PLACEMENT_3D('',#53451,#31129,#31130);
#26255=AXIS2_PLACEMENT_3D('',#53452,#31131,#31132);
#26256=AXIS2_PLACEMENT_3D('',#53453,#31133,#31134);
#26257=AXIS2_PLACEMENT_3D('',#53454,#31135,#31136);
#26258=AXIS2_PLACEMENT_3D('',#53455,#31137,#31138);
#26259=AXIS2_PLACEMENT_3D('',#53456,#31139,#31140);
#26260=AXIS2_PLACEMENT_3D('',#53457,#31141,#31142);
#26261=AXIS2_PLACEMENT_3D('',#53458,#31143,#31144);
#26262=AXIS2_PLACEMENT_3D('',#53459,#31145,#31146);
#26263=AXIS2_PLACEMENT_3D('',#53461,#31148,#31149);
#26264=AXIS2_PLACEMENT_3D('',#53463,#31151,#31152);
#26265=AXIS2_PLACEMENT_3D('',#53464,#31153,#31154);
#26266=AXIS2_PLACEMENT_3D('',#53465,#31155,#31156);
#26267=AXIS2_PLACEMENT_3D('',#53466,#31157,#31158);
#26268=AXIS2_PLACEMENT_3D('',#53467,#31159,#31160);
#30631=DIRECTION('axis',(0.,0.,1.));
#30632=DIRECTION('refdir',(1.,0.,0.));
#30633=DIRECTION('center_axis',(1.,0.,-3.96508223080413E-16));
#30634=DIRECTION('ref_axis',(-3.96508223080413E-16,0.,-1.));
#30635=DIRECTION('',(3.96508223080413E-16,0.,1.));
#30636=DIRECTION('',(0.,-1.,0.));
#30637=DIRECTION('',(3.96508223080413E-16,0.,1.));
#30638=DIRECTION('',(0.,-1.,0.));
#30639=DIRECTION('center_axis',(0.270745576918284,0.,-0.962650940153899));
#30640=DIRECTION('ref_axis',(-0.962650940153899,0.,-0.270745576918284));
#30641=DIRECTION('',(0.962650940153899,0.,0.270745576918284));
#30642=DIRECTION('',(0.,-1.,0.));
#30643=DIRECTION('',(0.962650940153899,0.,0.270745576918284));
#30644=DIRECTION('center_axis',(0.,0.,-1.));
#30645=DIRECTION('ref_axis',(-1.,0.,0.));
#30646=DIRECTION('',(1.,0.,0.));
#30647=DIRECTION('',(0.,-1.,0.));
#30648=DIRECTION('',(1.,0.,0.));
#30649=DIRECTION('center_axis',(1.,0.,0.));
#30650=DIRECTION('ref_axis',(0.,0.,-1.));
#30651=DIRECTION('',(0.,0.,1.));
#30652=DIRECTION('',(0.,-1.,0.));
#30653=DIRECTION('',(0.,0.,1.));
#30654=DIRECTION('center_axis',(0.,0.,-1.));
#30655=DIRECTION('ref_axis',(-1.,0.,0.));
#30656=DIRECTION('',(1.,0.,0.));
#30657=DIRECTION('',(1.,0.,0.));
#30658=DIRECTION('center_axis',(0.,1.,0.));
#30659=DIRECTION('ref_axis',(0.,0.,1.));
#30660=DIRECTION('center_axis',(0.,1.,0.));
#30661=DIRECTION('ref_axis',(0.,0.,1.));
#30662=DIRECTION('center_axis',(1.,0.,-3.96508223080413E-16));
#30663=DIRECTION('ref_axis',(-3.96508223080413E-16,0.,-1.));
#30664=DIRECTION('',(3.96508223080413E-16,0.,1.));
#30665=DIRECTION('',(0.,1.,0.));
#30666=DIRECTION('',(3.96508223080413E-16,0.,1.));
#30667=DIRECTION('',(0.,1.,0.));
#30668=DIRECTION('center_axis',(0.270745576918284,0.,-0.962650940153899));
#30669=DIRECTION('ref_axis',(-0.962650940153899,0.,-0.270745576918284));
#30670=DIRECTION('',(0.962650940153899,0.,0.270745576918284));
#30671=DIRECTION('',(0.962650940153899,0.,0.270745576918284));
#30672=DIRECTION('',(0.,1.,0.));
#30673=DIRECTION('center_axis',(0.,0.,-1.));
#30674=DIRECTION('ref_axis',(-1.,0.,0.));
#30675=DIRECTION('',(1.,0.,0.));
#30676=DIRECTION('',(1.,0.,0.));
#30677=DIRECTION('',(0.,1.,0.));
#30678=DIRECTION('center_axis',(1.,0.,0.));
#30679=DIRECTION('ref_axis',(0.,0.,-1.));
#30680=DIRECTION('',(0.,0.,1.));
#30681=DIRECTION('',(0.,0.,1.));
#30682=DIRECTION('',(0.,1.,0.));
#30683=DIRECTION('center_axis',(0.,0.,-1.));
#30684=DIRECTION('ref_axis',(-1.,0.,0.));
#30685=DIRECTION('',(1.,0.,0.));
#30686=DIRECTION('',(1.,0.,0.));
#30687=DIRECTION('center_axis',(0.,-1.,0.));
#30688=DIRECTION('ref_axis',(0.,0.,1.));
#30689=DIRECTION('center_axis',(0.,-1.,0.));
#30690=DIRECTION('ref_axis',(0.,0.,1.));
#30691=DIRECTION('center_axis',(0.,0.,-1.));
#30692=DIRECTION('ref_axis',(-1.,0.,0.));
#30693=DIRECTION('center_axis',(0.,0.,1.));
#30694=DIRECTION('ref_axis',(-1.,1.77635683940025E-15,0.));
#30695=DIRECTION('',(0.,0.,-1.));
#30696=DIRECTION('center_axis',(0.,0.,-1.));
#30697=DIRECTION('ref_axis',(-1.,0.,0.));
#30698=DIRECTION('',(0.,0.,-1.));
#30699=DIRECTION('center_axis',(0.,0.,1.));
#30700=DIRECTION('ref_axis',(1.,0.,0.));
#30701=DIRECTION('center_axis',(0.,0.,-1.));
#30702=DIRECTION('ref_axis',(-1.,0.,0.));
#30703=DIRECTION('',(0.,0.,1.));
#30704=DIRECTION('center_axis',(0.,0.,1.));
#30705=DIRECTION('ref_axis',(1.,0.,0.));
#30706=DIRECTION('center_axis',(0.,0.,1.));
#30707=DIRECTION('ref_axis',(1.,0.,0.));
#30708=DIRECTION('center_axis',(0.,0.,-1.));
#30709=DIRECTION('ref_axis',(-1.,0.,0.));
#30710=DIRECTION('',(0.,0.,1.));
#30711=DIRECTION('center_axis',(0.,0.,1.));
#30712=DIRECTION('ref_axis',(1.,0.,0.));
#30713=DIRECTION('center_axis',(0.,0.,1.));
#30714=DIRECTION('ref_axis',(1.,0.,0.));
#30715=DIRECTION('center_axis',(0.,0.,-1.));
#30716=DIRECTION('ref_axis',(-1.,0.,0.));
#30717=DIRECTION('',(0.,0.,1.));
#30718=DIRECTION('center_axis',(0.,0.,1.));
#30719=DIRECTION('ref_axis',(1.,0.,0.));
#30720=DIRECTION('center_axis',(0.,0.,1.));
#30721=DIRECTION('ref_axis',(1.,0.,0.));
#30722=DIRECTION('center_axis',(0.,0.,-1.));
#30723=DIRECTION('ref_axis',(-1.,0.,0.));
#30724=DIRECTION('',(0.,0.,1.));
#30725=DIRECTION('center_axis',(0.,0.,1.));
#30726=DIRECTION('ref_axis',(1.,0.,0.));
#30727=DIRECTION('center_axis',(0.,0.,1.));
#30728=DIRECTION('ref_axis',(1.,0.,0.));
#30729=DIRECTION('center_axis',(0.,0.,-1.));
#30730=DIRECTION('ref_axis',(-1.,0.,0.));
#30731=DIRECTION('',(0.,0.,1.));
#30732=DIRECTION('center_axis',(0.,0.,1.));
#30733=DIRECTION('ref_axis',(1.,0.,0.));
#30734=DIRECTION('center_axis',(0.,0.,1.));
#30735=DIRECTION('ref_axis',(1.,0.,0.));
#30736=DIRECTION('center_axis',(0.,0.,-1.));
#30737=DIRECTION('ref_axis',(-1.,0.,0.));
#30738=DIRECTION('',(0.,0.,1.));
#30739=DIRECTION('center_axis',(0.,0.,1.));
#30740=DIRECTION('ref_axis',(1.,0.,0.));
#30741=DIRECTION('center_axis',(0.,0.,1.));
#30742=DIRECTION('ref_axis',(1.,0.,0.));
#30743=DIRECTION('center_axis',(0.,0.,-1.));
#30744=DIRECTION('ref_axis',(-1.,0.,0.));
#30745=DIRECTION('',(0.,0.,1.));
#30746=DIRECTION('center_axis',(0.,0.,1.));
#30747=DIRECTION('ref_axis',(1.,0.,0.));
#30748=DIRECTION('center_axis',(0.,0.,1.));
#30749=DIRECTION('ref_axis',(1.,0.,0.));
#30750=DIRECTION('center_axis',(0.,0.,-1.));
#30751=DIRECTION('ref_axis',(-1.,0.,0.));
#30752=DIRECTION('',(0.,0.,1.));
#30753=DIRECTION('center_axis',(0.,0.,1.));
#30754=DIRECTION('ref_axis',(1.,0.,0.));
#30755=DIRECTION('center_axis',(0.,0.,1.));
#30756=DIRECTION('ref_axis',(1.,0.,0.));
#30757=DIRECTION('center_axis',(0.,0.,-1.));
#30758=DIRECTION('ref_axis',(-1.,0.,0.));
#30759=DIRECTION('',(0.,0.,1.));
#30760=DIRECTION('center_axis',(0.,0.,1.));
#30761=DIRECTION('ref_axis',(1.,0.,0.));
#30762=DIRECTION('center_axis',(0.,0.,1.));
#30763=DIRECTION('ref_axis',(1.,0.,0.));
#30764=DIRECTION('center_axis',(0.,0.,1.));
#30765=DIRECTION('ref_axis',(1.,0.,0.));
#30766=DIRECTION('',(0.,0.,1.));
#30767=DIRECTION('center_axis',(0.,0.,1.));
#30768=DIRECTION('ref_axis',(1.,0.,0.));
#30769=DIRECTION('center_axis',(-1.,0.,0.));
#30770=DIRECTION('ref_axis',(0.,0.,1.));
#30771=DIRECTION('center_axis',(1.,0.,0.));
#30772=DIRECTION('ref_axis',(0.,0.,-1.));
#30773=DIRECTION('',(-1.,0.,0.));
#30774=DIRECTION('center_axis',(-1.,0.,0.));
#30775=DIRECTION('ref_axis',(0.,0.,1.));
#30776=DIRECTION('center_axis',(-1.,0.,0.));
#30777=DIRECTION('ref_axis',(0.,0.,1.));
#30778=DIRECTION('center_axis',(1.,0.,0.));
#30779=DIRECTION('ref_axis',(0.,0.,-1.));
#30780=DIRECTION('',(-1.,0.,0.));
#30781=DIRECTION('center_axis',(-1.,0.,0.));
#30782=DIRECTION('ref_axis',(0.,0.,1.));
#30783=DIRECTION('center_axis',(-1.,0.,0.));
#30784=DIRECTION('ref_axis',(0.,0.,1.));
#30785=DIRECTION('center_axis',(1.,0.,0.));
#30786=DIRECTION('ref_axis',(0.,0.,-1.));
#30787=DIRECTION('',(-1.,0.,0.));
#30788=DIRECTION('center_axis',(-1.,0.,0.));
#30789=DIRECTION('ref_axis',(0.,0.,1.));
#30790=DIRECTION('center_axis',(-1.,0.,0.));
#30791=DIRECTION('ref_axis',(0.,0.,1.));
#30792=DIRECTION('center_axis',(1.,0.,0.));
#30793=DIRECTION('ref_axis',(0.,0.,-1.));
#30794=DIRECTION('',(-1.,0.,0.));
#30795=DIRECTION('center_axis',(-1.,0.,0.));
#30796=DIRECTION('ref_axis',(0.,0.,1.));
#30797=DIRECTION('center_axis',(-1.,0.,0.));
#30798=DIRECTION('ref_axis',(0.,0.,1.));
#30799=DIRECTION('center_axis',(1.,0.,0.));
#30800=DIRECTION('ref_axis',(0.,0.,-1.));
#30801=DIRECTION('',(-1.,0.,0.));
#30802=DIRECTION('center_axis',(-1.,0.,0.));
#30803=DIRECTION('ref_axis',(0.,0.,1.));
#30804=DIRECTION('center_axis',(-1.,0.,0.));
#30805=DIRECTION('ref_axis',(0.,0.,1.));
#30806=DIRECTION('center_axis',(1.,0.,0.));
#30807=DIRECTION('ref_axis',(0.,0.,-1.));
#30808=DIRECTION('',(-1.,0.,0.));
#30809=DIRECTION('center_axis',(-1.,0.,0.));
#30810=DIRECTION('ref_axis',(0.,0.,1.));
#30811=DIRECTION('center_axis',(1.,0.,0.));
#30812=DIRECTION('ref_axis',(0.,0.,-1.));
#30813=DIRECTION('center_axis',(1.,0.,0.));
#30814=DIRECTION('ref_axis',(0.,0.,-1.));
#30815=DIRECTION('',(1.,0.,0.));
#30816=DIRECTION('center_axis',(1.,0.,0.));
#30817=DIRECTION('ref_axis',(0.,0.,-1.));
#30818=DIRECTION('center_axis',(1.,0.,0.));
#30819=DIRECTION('ref_axis',(0.,0.,-1.));
#30820=DIRECTION('center_axis',(1.,0.,0.));
#30821=DIRECTION('ref_axis',(0.,0.,-1.));
#30822=DIRECTION('',(1.,0.,0.));
#30823=DIRECTION('center_axis',(1.,0.,0.));
#30824=DIRECTION('ref_axis',(0.,0.,-1.));
#30825=DIRECTION('center_axis',(1.,0.,0.));
#30826=DIRECTION('ref_axis',(0.,0.,-1.));
#30827=DIRECTION('center_axis',(1.,0.,0.));
#30828=DIRECTION('ref_axis',(0.,0.,-1.));
#30829=DIRECTION('',(1.,0.,0.));
#30830=DIRECTION('center_axis',(1.,0.,0.));
#30831=DIRECTION('ref_axis',(0.,0.,-1.));
#30832=DIRECTION('center_axis',(1.,0.,0.));
#30833=DIRECTION('ref_axis',(0.,0.,-1.));
#30834=DIRECTION('center_axis',(1.,0.,0.));
#30835=DIRECTION('ref_axis',(0.,0.,-1.));
#30836=DIRECTION('',(1.,0.,0.));
#30837=DIRECTION('center_axis',(1.,0.,0.));
#30838=DIRECTION('ref_axis',(0.,0.,-1.));
#30839=DIRECTION('center_axis',(1.,0.,0.));
#30840=DIRECTION('ref_axis',(0.,0.,-1.));
#30841=DIRECTION('center_axis',(1.,0.,0.));
#30842=DIRECTION('ref_axis',(0.,0.,-1.));
#30843=DIRECTION('',(1.,0.,0.));
#30844=DIRECTION('center_axis',(1.,0.,0.));
#30845=DIRECTION('ref_axis',(0.,0.,-1.));
#30846=DIRECTION('center_axis',(1.,0.,0.));
#30847=DIRECTION('ref_axis',(0.,0.,-1.));
#30848=DIRECTION('center_axis',(1.,0.,0.));
#30849=DIRECTION('ref_axis',(0.,0.,-1.));
#30850=DIRECTION('',(1.,0.,0.));
#30851=DIRECTION('center_axis',(1.,0.,0.));
#30852=DIRECTION('ref_axis',(0.,0.,-1.));
#30853=DIRECTION('center_axis',(1.,0.,0.));
#30854=DIRECTION('ref_axis',(0.,0.,-1.));
#30855=DIRECTION('center_axis',(1.,0.,0.));
#30856=DIRECTION('ref_axis',(0.,0.,-1.));
#30857=DIRECTION('',(1.,0.,0.));
#30858=DIRECTION('center_axis',(1.,0.,0.));
#30859=DIRECTION('ref_axis',(0.,0.,-1.));
#30860=DIRECTION('center_axis',(1.,0.,0.));
#30861=DIRECTION('ref_axis',(0.,0.,-1.));
#30862=DIRECTION('center_axis',(1.,0.,0.));
#30863=DIRECTION('ref_axis',(0.,0.,-1.));
#30864=DIRECTION('',(1.,0.,0.));
#30865=DIRECTION('center_axis',(1.,0.,0.));
#30866=DIRECTION('ref_axis',(0.,0.,-1.));
#30867=DIRECTION('center_axis',(1.,0.,0.));
#30868=DIRECTION('ref_axis',(0.,0.,-1.));
#30869=DIRECTION('center_axis',(1.,0.,0.));
#30870=DIRECTION('ref_axis',(0.,0.,-1.));
#30871=DIRECTION('',(1.,0.,0.));
#30872=DIRECTION('center_axis',(1.,0.,0.));
#30873=DIRECTION('ref_axis',(0.,0.,-1.));
#30874=DIRECTION('center_axis',(1.,0.,0.));
#30875=DIRECTION('ref_axis',(0.,0.,-1.));
#30876=DIRECTION('center_axis',(1.,0.,0.));
#30877=DIRECTION('ref_axis',(0.,0.,-1.));
#30878=DIRECTION('',(1.,0.,0.));
#30879=DIRECTION('center_axis',(1.,0.,0.));
#30880=DIRECTION('ref_axis',(0.,0.,-1.));
#30881=DIRECTION('center_axis',(1.,0.,0.));
#30882=DIRECTION('ref_axis',(0.,0.,-1.));
#30883=DIRECTION('center_axis',(1.,0.,0.));
#30884=DIRECTION('ref_axis',(0.,0.,-1.));
#30885=DIRECTION('',(1.,0.,0.));
#30886=DIRECTION('center_axis',(1.,0.,0.));
#30887=DIRECTION('ref_axis',(0.,0.,-1.));
#30888=DIRECTION('center_axis',(1.,0.,0.));
#30889=DIRECTION('ref_axis',(0.,0.,-1.));
#30890=DIRECTION('center_axis',(1.,0.,0.));
#30891=DIRECTION('ref_axis',(0.,0.,-1.));
#30892=DIRECTION('',(1.,0.,0.));
#30893=DIRECTION('center_axis',(1.,0.,0.));
#30894=DIRECTION('ref_axis',(0.,0.,-1.));
#30895=DIRECTION('center_axis',(1.,0.,0.));
#30896=DIRECTION('ref_axis',(0.,0.,-1.));
#30897=DIRECTION('center_axis',(1.,0.,0.));
#30898=DIRECTION('ref_axis',(0.,0.,-1.));
#30899=DIRECTION('',(1.,0.,0.));
#30900=DIRECTION('center_axis',(1.,0.,0.));
#30901=DIRECTION('ref_axis',(0.,0.,-1.));
#30902=DIRECTION('center_axis',(1.,0.,0.));
#30903=DIRECTION('ref_axis',(0.,0.,-1.));
#30904=DIRECTION('center_axis',(1.,0.,0.));
#30905=DIRECTION('ref_axis',(0.,0.,-1.));
#30906=DIRECTION('',(1.,0.,0.));
#30907=DIRECTION('center_axis',(1.,0.,0.));
#30908=DIRECTION('ref_axis',(0.,0.,-1.));
#30909=DIRECTION('center_axis',(1.,0.,0.));
#30910=DIRECTION('ref_axis',(0.,0.,-1.));
#30911=DIRECTION('center_axis',(1.,0.,0.));
#30912=DIRECTION('ref_axis',(0.,0.,-1.));
#30913=DIRECTION('',(1.,0.,0.));
#30914=DIRECTION('center_axis',(1.,0.,0.));
#30915=DIRECTION('ref_axis',(0.,0.,-1.));
#30916=DIRECTION('center_axis',(1.,0.,0.));
#30917=DIRECTION('ref_axis',(0.,0.,-1.));
#30918=DIRECTION('center_axis',(1.,0.,0.));
#30919=DIRECTION('ref_axis',(0.,0.,-1.));
#30920=DIRECTION('',(1.,0.,0.));
#30921=DIRECTION('center_axis',(1.,0.,0.));
#30922=DIRECTION('ref_axis',(0.,0.,-1.));
#30923=DIRECTION('center_axis',(1.,0.,0.));
#30924=DIRECTION('ref_axis',(0.,0.,-1.));
#30925=DIRECTION('center_axis',(1.,0.,0.));
#30926=DIRECTION('ref_axis',(0.,0.,-1.));
#30927=DIRECTION('',(1.,0.,0.));
#30928=DIRECTION('center_axis',(1.,0.,0.));
#30929=DIRECTION('ref_axis',(0.,0.,-1.));
#30930=DIRECTION('center_axis',(1.,0.,0.));
#30931=DIRECTION('ref_axis',(0.,0.,-1.));
#30932=DIRECTION('center_axis',(1.,0.,0.));
#30933=DIRECTION('ref_axis',(0.,0.,-1.));
#30934=DIRECTION('',(1.,0.,0.));
#30935=DIRECTION('center_axis',(1.,0.,0.));
#30936=DIRECTION('ref_axis',(0.,0.,-1.));
#30937=DIRECTION('center_axis',(1.,0.,0.));
#30938=DIRECTION('ref_axis',(0.,0.,-1.));
#30939=DIRECTION('center_axis',(1.,0.,0.));
#30940=DIRECTION('ref_axis',(0.,0.,-1.));
#30941=DIRECTION('',(1.,0.,0.));
#30942=DIRECTION('center_axis',(1.,0.,0.));
#30943=DIRECTION('ref_axis',(0.,0.,-1.));
#30944=DIRECTION('center_axis',(1.,0.,0.));
#30945=DIRECTION('ref_axis',(0.,0.,-1.));
#30946=DIRECTION('center_axis',(1.,0.,0.));
#30947=DIRECTION('ref_axis',(0.,0.,-1.));
#30948=DIRECTION('',(1.,0.,0.));
#30949=DIRECTION('center_axis',(1.,0.,0.));
#30950=DIRECTION('ref_axis',(0.,0.,-1.));
#30951=DIRECTION('center_axis',(1.,0.,0.));
#30952=DIRECTION('ref_axis',(0.,0.,-1.));
#30953=DIRECTION('center_axis',(1.,0.,0.));
#30954=DIRECTION('ref_axis',(0.,0.,-1.));
#30955=DIRECTION('',(1.,0.,0.));
#30956=DIRECTION('center_axis',(1.,0.,0.));
#30957=DIRECTION('ref_axis',(0.,0.,-1.));
#30958=DIRECTION('center_axis',(1.,0.,0.));
#30959=DIRECTION('ref_axis',(0.,0.,-1.));
#30960=DIRECTION('center_axis',(1.,0.,0.));
#30961=DIRECTION('ref_axis',(0.,0.,-1.));
#30962=DIRECTION('',(1.,0.,0.));
#30963=DIRECTION('center_axis',(1.,0.,0.));
#30964=DIRECTION('ref_axis',(0.,0.,-1.));
#30965=DIRECTION('center_axis',(1.,0.,0.));
#30966=DIRECTION('ref_axis',(0.,0.,-1.));
#30967=DIRECTION('center_axis',(1.,0.,0.));
#30968=DIRECTION('ref_axis',(0.,0.,-1.));
#30969=DIRECTION('',(1.,0.,0.));
#30970=DIRECTION('center_axis',(1.,0.,0.));
#30971=DIRECTION('ref_axis',(0.,0.,-1.));
#30972=DIRECTION('center_axis',(1.,0.,0.));
#30973=DIRECTION('ref_axis',(0.,0.,-1.));
#30974=DIRECTION('center_axis',(1.,0.,0.));
#30975=DIRECTION('ref_axis',(0.,0.,-1.));
#30976=DIRECTION('',(1.,0.,0.));
#30977=DIRECTION('center_axis',(1.,0.,0.));
#30978=DIRECTION('ref_axis',(0.,0.,-1.));
#30979=DIRECTION('center_axis',(1.,0.,0.));
#30980=DIRECTION('ref_axis',(0.,0.,-1.));
#30981=DIRECTION('center_axis',(1.,0.,0.));
#30982=DIRECTION('ref_axis',(0.,0.,-1.));
#30983=DIRECTION('',(1.,0.,0.));
#30984=DIRECTION('center_axis',(1.,0.,0.));
#30985=DIRECTION('ref_axis',(0.,0.,-1.));
#30986=DIRECTION('center_axis',(1.,0.,0.));
#30987=DIRECTION('ref_axis',(0.,0.,-1.));
#30988=DIRECTION('center_axis',(1.,0.,0.));
#30989=DIRECTION('ref_axis',(0.,0.,-1.));
#30990=DIRECTION('',(1.,0.,0.));
#30991=DIRECTION('center_axis',(1.,0.,0.));
#30992=DIRECTION('ref_axis',(0.,0.,-1.));
#30993=DIRECTION('center_axis',(1.,0.,0.));
#30994=DIRECTION('ref_axis',(0.,0.,-1.));
#30995=DIRECTION('center_axis',(1.,0.,0.));
#30996=DIRECTION('ref_axis',(0.,0.,-1.));
#30997=DIRECTION('',(1.,0.,0.));
#30998=DIRECTION('center_axis',(1.,0.,0.));
#30999=DIRECTION('ref_axis',(0.,0.,-1.));
#31000=DIRECTION('center_axis',(1.,0.,0.));
#31001=DIRECTION('ref_axis',(0.,0.,-1.));
#31002=DIRECTION('center_axis',(1.,0.,0.));
#31003=DIRECTION('ref_axis',(0.,0.,-1.));
#31004=DIRECTION('',(1.,0.,0.));
#31005=DIRECTION('center_axis',(1.,0.,0.));
#31006=DIRECTION('ref_axis',(0.,0.,-1.));
#31007=DIRECTION('center_axis',(1.,0.,0.));
#31008=DIRECTION('ref_axis',(0.,0.,-1.));
#31009=DIRECTION('center_axis',(1.,0.,0.));
#31010=DIRECTION('ref_axis',(0.,0.,-1.));
#31011=DIRECTION('',(1.,0.,0.));
#31012=DIRECTION('center_axis',(1.,0.,0.));
#31013=DIRECTION('ref_axis',(0.,0.,-1.));
#31014=DIRECTION('center_axis',(1.,0.,0.));
#31015=DIRECTION('ref_axis',(0.,0.,-1.));
#31016=DIRECTION('center_axis',(1.,0.,0.));
#31017=DIRECTION('ref_axis',(0.,0.,-1.));
#31018=DIRECTION('',(1.,0.,0.));
#31019=DIRECTION('center_axis',(1.,0.,0.));
#31020=DIRECTION('ref_axis',(0.,0.,-1.));
#31021=DIRECTION('center_axis',(1.,0.,0.));
#31022=DIRECTION('ref_axis',(0.,0.,-1.));
#31023=DIRECTION('center_axis',(1.,0.,0.));
#31024=DIRECTION('ref_axis',(0.,0.,-1.));
#31025=DIRECTION('',(1.,0.,0.));
#31026=DIRECTION('center_axis',(1.,0.,0.));
#31027=DIRECTION('ref_axis',(0.,0.,-1.));
#31028=DIRECTION('center_axis',(1.,0.,0.));
#31029=DIRECTION('ref_axis',(0.,0.,-1.));
#31030=DIRECTION('center_axis',(1.,0.,0.));
#31031=DIRECTION('ref_axis',(0.,0.,-1.));
#31032=DIRECTION('',(1.,0.,0.));
#31033=DIRECTION('center_axis',(1.,0.,0.));
#31034=DIRECTION('ref_axis',(0.,0.,-1.));
#31035=DIRECTION('center_axis',(-1.,-1.73472347597681E-16,0.));
#31036=DIRECTION('ref_axis',(1.73472347597681E-16,-1.,0.));
#31037=DIRECTION('',(0.,1.,1.18952466924124E-16));
#31038=DIRECTION('',(1.2266347333467E-16,-0.707106781186546,0.707106781186549));
#31039=DIRECTION('',(0.,1.26161707343768E-16,-1.));
#31040=DIRECTION('',(-1.2266347333467E-16,0.70710678118655,0.707106781186545));
#31041=DIRECTION('',(0.,-1.,-1.58603289232165E-16));
#31042=DIRECTION('',(-1.2266347333467E-16,0.707106781186546,-0.707106781186548));
#31043=DIRECTION('',(0.,0.,1.));
#31044=DIRECTION('',(1.2266347333467E-16,-0.70710678118655,-0.707106781186545));
#31045=DIRECTION('center_axis',(0.,1.,0.));
#31046=DIRECTION('ref_axis',(0.,0.,1.));
#31047=DIRECTION('',(1.,0.,0.));
#31048=DIRECTION('',(0.,0.,1.));
#31049=DIRECTION('',(1.,0.,0.));
#31050=DIRECTION('',(0.,0.,-1.));
#31051=DIRECTION('center_axis',(-1.,0.,0.));
#31052=DIRECTION('ref_axis',(0.,0.,1.));
#31053=DIRECTION('',(0.,1.,0.));
#31054=DIRECTION('',(0.,0.,-1.));
#31055=DIRECTION('',(0.,1.,0.));
#31056=DIRECTION('',(0.,0.,1.));
#31057=DIRECTION('center_axis',(0.,1.,0.));
#31058=DIRECTION('ref_axis',(0.,0.,1.));
#31059=DIRECTION('',(1.,0.,0.));
#31060=DIRECTION('',(0.,0.,-1.));
#31061=DIRECTION('',(1.,0.,0.));
#31062=DIRECTION('',(0.,0.,-1.));
#31063=DIRECTION('center_axis',(0.,0.,-1.));
#31064=DIRECTION('ref_axis',(-1.,0.,0.));
#31065=DIRECTION('',(0.707106781186548,0.707106781186547,0.));
#31066=DIRECTION('',(-0.707106781186546,0.707106781186549,0.));
#31067=DIRECTION('',(0.,-1.,0.));
#31068=DIRECTION('',(1.,0.,0.));
#31069=DIRECTION('',(-1.,0.,0.));
#31070=DIRECTION('center_axis',(0.,0.,1.));
#31071=DIRECTION('ref_axis',(-1.,0.,0.));
#31072=DIRECTION('center_axis',(0.,0.,-1.));
#31073=DIRECTION('ref_axis',(-1.,0.,0.));
#31074=DIRECTION('',(-0.707106781186548,-0.707106781186547,0.));
#31075=DIRECTION('',(0.,-1.,0.));
#31076=DIRECTION('',(0.707106781186546,-0.707106781186549,0.));
#31077=DIRECTION('',(-1.,0.,0.));
#31078=DIRECTION('center_axis',(0.,0.,-1.));
#31079=DIRECTION('ref_axis',(-1.,0.,0.));
#31080=DIRECTION('',(1.,0.,0.));
#31081=DIRECTION('center_axis',(1.,0.,0.));
#31082=DIRECTION('ref_axis',(0.,0.,-1.));
#31083=DIRECTION('',(0.,1.26161707343768E-16,-1.));
#31084=DIRECTION('',(0.,0.707106781186546,-0.707106781186549));
#31085=DIRECTION('',(0.,1.,1.18952466924124E-16));
#31086=DIRECTION('',(0.,0.70710678118655,0.707106781186545));
#31087=DIRECTION('',(0.,0.,1.));
#31088=DIRECTION('',(0.,-0.707106781186546,0.707106781186548));
#31089=DIRECTION('',(0.,-1.,-1.58603289232165E-16));
#31090=DIRECTION('',(0.,-0.70710678118655,-0.707106781186545));
#31091=DIRECTION('center_axis',(0.,-1.18952466924124E-16,1.));
#31092=DIRECTION('ref_axis',(0.,-1.,-1.18952466924124E-16));
#31093=DIRECTION('',(-1.,0.,0.));
#31094=DIRECTION('',(1.,0.,0.));
#31095=DIRECTION('center_axis',(0.,-1.,0.));
#31096=DIRECTION('ref_axis',(0.,0.,-1.));
#31097=DIRECTION('',(1.,0.,0.));
#31098=DIRECTION('',(-1.,0.,0.));
#31099=DIRECTION('center_axis',(0.,1.58603289232165E-16,-1.));
#31100=DIRECTION('ref_axis',(0.,1.,1.58603289232165E-16));
#31101=DIRECTION('',(1.,0.,0.));
#31102=DIRECTION('',(-1.,0.,0.));
#31103=DIRECTION('center_axis',(0.,1.,1.26161707343768E-16));
#31104=DIRECTION('ref_axis',(0.,-1.26161707343768E-16,1.));
#31105=DIRECTION('',(1.,0.,0.));
#31106=DIRECTION('',(-1.,0.,0.));
#31107=DIRECTION('center_axis',(-1.,0.,0.));
#31108=DIRECTION('ref_axis',(0.,0.,1.));
#31109=DIRECTION('center_axis',(-1.,0.,0.));
#31110=DIRECTION('ref_axis',(0.,0.,1.));
#31111=DIRECTION('center_axis',(-1.,0.,0.));
#31112=DIRECTION('ref_axis',(0.,0.,1.));
#31113=DIRECTION('center_axis',(-1.,0.,0.));
#31114=DIRECTION('ref_axis',(0.,0.,1.));
#31115=DIRECTION('center_axis',(-1.,0.,0.));
#31116=DIRECTION('ref_axis',(0.,0.,1.));
#31117=DIRECTION('center_axis',(-1.,0.,0.));
#31118=DIRECTION('ref_axis',(0.,0.,1.));
#31119=DIRECTION('center_axis',(-1.,0.,0.));
#31120=DIRECTION('ref_axis',(0.,0.,1.));
#31121=DIRECTION('center_axis',(-1.,0.,0.));
#31122=DIRECTION('ref_axis',(0.,0.,1.));
#31123=DIRECTION('center_axis',(-1.,0.,0.));
#31124=DIRECTION('ref_axis',(0.,0.,1.));
#31125=DIRECTION('center_axis',(-1.,0.,0.));
#31126=DIRECTION('ref_axis',(0.,0.,1.));
#31127=DIRECTION('center_axis',(-1.,0.,0.));
#31128=DIRECTION('ref_axis',(0.,0.,1.));
#31129=DIRECTION('center_axis',(-1.,0.,0.));
#31130=DIRECTION('ref_axis',(0.,0.,1.));
#31131=DIRECTION('center_axis',(-1.,0.,0.));
#31132=DIRECTION('ref_axis',(0.,0.,1.));
#31133=DIRECTION('center_axis',(-1.,0.,0.));
#31134=DIRECTION('ref_axis',(0.,0.,1.));
#31135=DIRECTION('center_axis',(-1.,0.,0.));
#31136=DIRECTION('ref_axis',(0.,0.,1.));
#31137=DIRECTION('center_axis',(-1.,0.,0.));
#31138=DIRECTION('ref_axis',(0.,0.,1.));
#31139=DIRECTION('center_axis',(0.,0.,1.));
#31140=DIRECTION('ref_axis',(1.,0.,0.));
#31141=DIRECTION('center_axis',(-0.707106781186547,0.707106781186548,0.));
#31142=DIRECTION('ref_axis',(0.,0.,-1.));
#31143=DIRECTION('center_axis',(0.707106781186549,0.707106781186546,0.));
#31144=DIRECTION('ref_axis',(0.,0.,1.));
#31145=DIRECTION('center_axis',(0.,-1.,0.));
#31146=DIRECTION('ref_axis',(0.,0.,-1.));
#31147=DIRECTION('',(0.,0.,-1.));
#31148=DIRECTION('center_axis',(0.,1.,0.));
#31149=DIRECTION('ref_axis',(0.,0.,1.));
#31150=DIRECTION('',(0.,0.,-1.));
#31151=DIRECTION('center_axis',(0.,0.,-1.));
#31152=DIRECTION('ref_axis',(1.,1.22464679914735E-16,0.));
#31153=DIRECTION('center_axis',(0.,0.707106781186549,0.707106781186546));
#31154=DIRECTION('ref_axis',(-1.,0.,0.));
#31155=DIRECTION('center_axis',(0.,0.707106781186545,-0.70710678118655));
#31156=DIRECTION('ref_axis',(-1.,0.,0.));
#31157=DIRECTION('center_axis',(0.,-0.707106781186549,-0.707106781186547));
#31158=DIRECTION('ref_axis',(-1.,0.,0.));
#31159=DIRECTION('center_axis',(0.,-0.707106781186545,0.70710678118655));
#31160=DIRECTION('ref_axis',(-1.,0.,0.));
#52987=CARTESIAN_POINT('',(0.,0.,0.));
#52988=CARTESIAN_POINT('Origin',(-113.,125.,4.48054292080867E-14));
#52989=CARTESIAN_POINT('',(-113.,115.,-41.));
#52990=CARTESIAN_POINT('',(-113.,115.,-6.));
#52991=CARTESIAN_POINT('',(-113.,115.,4.48054292080867E-14));
#52992=CARTESIAN_POINT('',(-113.,125.,-41.));
#52993=CARTESIAN_POINT('',(-113.,125.,-41.));
#52994=CARTESIAN_POINT('',(-113.,125.,-6.));
#52995=CARTESIAN_POINT('',(-113.,125.,4.48054292080867E-14));
#52996=CARTESIAN_POINT('',(-113.,125.,-6.));
#52997=CARTESIAN_POINT('Origin',(2.4027149321267,125.,-8.54298642533938));
#52998=CARTESIAN_POINT('',(-273.,115.,-86.));
#52999=CARTESIAN_POINT('',(2.4027149321267,115.,-8.54298642533938));
#53000=CARTESIAN_POINT('',(-273.,125.,-86.));
#53001=CARTESIAN_POINT('',(-273.,125.,-86.));
#53002=CARTESIAN_POINT('',(2.4027149321267,125.,-8.54298642533938));
#53003=CARTESIAN_POINT('Origin',(0.,125.,-86.));
#53004=CARTESIAN_POINT('',(-308.,115.,-86.));
#53005=CARTESIAN_POINT('',(0.,115.,-86.));
#53006=CARTESIAN_POINT('',(-308.,125.,-86.));
#53007=CARTESIAN_POINT('',(-308.,125.,-86.));
#53008=CARTESIAN_POINT('',(0.,125.,-86.));
#53009=CARTESIAN_POINT('Origin',(-308.,125.,0.));
#53010=CARTESIAN_POINT('',(-308.,115.,-6.));
#53011=CARTESIAN_POINT('',(-308.,115.,0.));
#53012=CARTESIAN_POINT('',(-308.,125.,-6.));
#53013=CARTESIAN_POINT('',(-308.,125.,-6.));
#53014=CARTESIAN_POINT('',(-308.,125.,0.));
#53015=CARTESIAN_POINT('Origin',(0.,125.,-6.));
#53016=CARTESIAN_POINT('',(0.,115.,-6.));
#53017=CARTESIAN_POINT('',(0.,125.,-6.));
#53018=CARTESIAN_POINT('Origin',(0.,125.,0.));
#53019=CARTESIAN_POINT('Origin',(0.,115.,0.));
#53020=CARTESIAN_POINT('Origin',(-113.,-125.,4.48054292080867E-14));
#53021=CARTESIAN_POINT('',(-113.,-115.,-41.));
#53022=CARTESIAN_POINT('',(-113.,-115.,-6.));
#53023=CARTESIAN_POINT('',(-113.,-115.,4.48054292080867E-14));
#53024=CARTESIAN_POINT('',(-113.,-125.,-6.));
#53025=CARTESIAN_POINT('',(-113.,-125.,-6.));
#53026=CARTESIAN_POINT('',(-113.,-125.,-41.));
#53027=CARTESIAN_POINT('',(-113.,-125.,4.48054292080867E-14));
#53028=CARTESIAN_POINT('',(-113.,-125.,-41.));
#53029=CARTESIAN_POINT('Origin',(2.4027149321267,-125.,-8.54298642533938));
#53030=CARTESIAN_POINT('',(-273.,-115.,-86.));
#53031=CARTESIAN_POINT('',(2.4027149321267,-115.,-8.54298642533938));
#53032=CARTESIAN_POINT('',(-273.,-125.,-86.));
#53033=CARTESIAN_POINT('',(2.4027149321267,-125.,-8.54298642533938));
#53034=CARTESIAN_POINT('',(-273.,-125.,-86.));
#53035=CARTESIAN_POINT('Origin',(0.,-125.,-86.));
#53036=CARTESIAN_POINT('',(-308.,-115.,-86.));
#53037=CARTESIAN_POINT('',(0.,-115.,-86.));
#53038=CARTESIAN_POINT('',(-308.,-125.,-86.));
#53039=CARTESIAN_POINT('',(0.,-125.,-86.));
#53040=CARTESIAN_POINT('',(-308.,-125.,-86.));
#53041=CARTESIAN_POINT('Origin',(-308.,-125.,0.));
#53042=CARTESIAN_POINT('',(-308.,-115.,-6.));
#53043=CARTESIAN_POINT('',(-308.,-115.,0.));
#53044=CARTESIAN_POINT('',(-308.,-125.,-6.));
#53045=CARTESIAN_POINT('',(-308.,-125.,0.));
#53046=CARTESIAN_POINT('',(-308.,-125.,-6.));
#53047=CARTESIAN_POINT('Origin',(0.,-125.,-6.));
#53048=CARTESIAN_POINT('',(0.,-115.,-6.));
#53049=CARTESIAN_POINT('',(0.,-125.,-6.));
#53050=CARTESIAN_POINT('Origin',(0.,-125.,0.));
#53051=CARTESIAN_POINT('Origin',(0.,-115.,0.));
#53052=CARTESIAN_POINT('Origin',(2.5,2.75545529808155E-15,110.001));
#53053=CARTESIAN_POINT('',(2.50000000000002,55.,6.00000000000001));
#53054=CARTESIAN_POINT('',(2.50000000000001,-55.,6.00000000000001));
#53055=CARTESIAN_POINT('Origin',(2.5,2.75545529808155E-15,6.00000000000001));
#53056=CARTESIAN_POINT('',(2.50000000000001,-55.,-6.));
#53057=CARTESIAN_POINT('',(2.50000000000001,-55.,110.001));
#53058=CARTESIAN_POINT('',(2.50000000000002,55.,-6.));
#53059=CARTESIAN_POINT('Origin',(2.5,2.75545529808155E-15,-6.));
#53060=CARTESIAN_POINT('',(2.50000000000002,55.,110.001));
#53061=CARTESIAN_POINT('Origin',(-50.,47.5,6.));
#53062=CARTESIAN_POINT('',(-53.4,47.5,-6.));
#53063=CARTESIAN_POINT('Origin',(-50.,47.5,-6.));
#53064=CARTESIAN_POINT('',(-53.4,47.5,6.));
#53065=CARTESIAN_POINT('',(-53.4,47.5,6.));
#53066=CARTESIAN_POINT('Origin',(-50.,47.5,6.));
#53067=CARTESIAN_POINT('Origin',(70.,47.5,6.));
#53068=CARTESIAN_POINT('',(66.6,47.5,-6.));
#53069=CARTESIAN_POINT('Origin',(70.,47.5,-6.));
#53070=CARTESIAN_POINT('',(66.6,47.5,6.));
#53071=CARTESIAN_POINT('',(66.6,47.5,6.));
#53072=CARTESIAN_POINT('Origin',(70.,47.5,6.));
#53073=CARTESIAN_POINT('Origin',(70.,-47.5,6.));
#53074=CARTESIAN_POINT('',(66.6,-47.5,-6.));
#53075=CARTESIAN_POINT('Origin',(70.,-47.5,-6.));
#53076=CARTESIAN_POINT('',(66.6,-47.5,6.));
#53077=CARTESIAN_POINT('',(66.6,-47.5,6.));
#53078=CARTESIAN_POINT('Origin',(70.,-47.5,6.));
#53079=CARTESIAN_POINT('Origin',(-50.,-47.5,6.));
#53080=CARTESIAN_POINT('',(-53.4,-47.5,-6.));
#53081=CARTESIAN_POINT('Origin',(-50.,-47.5,-6.));
#53082=CARTESIAN_POINT('',(-53.4,-47.5,6.));
#53083=CARTESIAN_POINT('',(-53.4,-47.5,6.));
#53084=CARTESIAN_POINT('Origin',(-50.,-47.5,6.));
#53085=CARTESIAN_POINT('Origin',(-248.336309447889,58.3363094478911,6.));
#53086=CARTESIAN_POINT('',(-252.586309447889,58.3363094478911,-6.));
#53087=CARTESIAN_POINT('Origin',(-248.336309447889,58.3363094478911,-6.));
#53088=CARTESIAN_POINT('',(-252.586309447889,58.3363094478911,6.));
#53089=CARTESIAN_POINT('',(-252.586309447889,58.3363094478911,6.));
#53090=CARTESIAN_POINT('Origin',(-248.336309447889,58.3363094478911,6.));
#53091=CARTESIAN_POINT('Origin',(-248.33630944789,-58.3363094478899,6.));
#53092=CARTESIAN_POINT('',(-252.58630944789,-58.3363094478899,-6.));
#53093=CARTESIAN_POINT('Origin',(-248.33630944789,-58.3363094478899,-6.));
#53094=CARTESIAN_POINT('',(-252.58630944789,-58.3363094478899,6.));
#53095=CARTESIAN_POINT('',(-252.58630944789,-58.3363094478899,6.));
#53096=CARTESIAN_POINT('Origin',(-248.33630944789,-58.3363094478899,6.));
#53097=CARTESIAN_POINT('Origin',(-131.66369055211,-58.3363094478907,6.));
#53098=CARTESIAN_POINT('',(-135.91369055211,-58.3363094478907,-6.));
#53099=CARTESIAN_POINT('Origin',(-131.66369055211,-58.3363094478907,-6.));
#53100=CARTESIAN_POINT('',(-135.91369055211,-58.3363094478907,6.));
#53101=CARTESIAN_POINT('',(-135.91369055211,-58.3363094478907,6.));
#53102=CARTESIAN_POINT('Origin',(-131.66369055211,-58.3363094478907,6.));
#53103=CARTESIAN_POINT('Origin',(-131.66369055211,58.3363094478899,6.));
#53104=CARTESIAN_POINT('',(-135.91369055211,58.3363094478899,-6.));
#53105=CARTESIAN_POINT('Origin',(-131.66369055211,58.3363094478899,-6.));
#53106=CARTESIAN_POINT('',(-135.91369055211,58.3363094478899,6.));
#53107=CARTESIAN_POINT('',(-135.91369055211,58.3363094478899,6.));
#53108=CARTESIAN_POINT('Origin',(-131.66369055211,58.3363094478899,6.));
#53109=CARTESIAN_POINT('Origin',(-190.,0.,-110.));
#53110=CARTESIAN_POINT('',(-235.,-5.51091059616309E-15,-6.));
#53111=CARTESIAN_POINT('Origin',(-190.,0.,-6.00000000000001));
#53112=CARTESIAN_POINT('',(-235.,-5.51091059616309E-15,0.999999999999996));
#53113=CARTESIAN_POINT('',(-235.,-5.51091059616309E-15,-110.));
#53114=CARTESIAN_POINT('Origin',(-190.,0.,1.));
#53115=CARTESIAN_POINT('Origin',(-190.,0.,1.));
#53116=CARTESIAN_POINT('',(-255.,-7.9602041944578E-15,1.));
#53117=CARTESIAN_POINT('Origin',(-190.,0.,1.));
#53118=CARTESIAN_POINT('',(-255.,-7.9602041944578E-15,6.));
#53119=CARTESIAN_POINT('',(-255.,-7.9602041944578E-15,1.));
#53120=CARTESIAN_POINT('Origin',(-190.,0.,6.));
#53121=CARTESIAN_POINT('Origin',(-320.,13.9999999999999,-25.));
#53122=CARTESIAN_POINT('',(-308.,13.9999999999999,-28.));
#53123=CARTESIAN_POINT('Origin',(-308.,13.9999999999999,-25.));
#53124=CARTESIAN_POINT('',(-320.,13.9999999999999,-28.));
#53125=CARTESIAN_POINT('',(-320.,13.9999999999999,-28.));
#53126=CARTESIAN_POINT('Origin',(-320.,13.9999999999999,-25.));
#53127=CARTESIAN_POINT('Origin',(-320.,-14.0000000000001,25.));
#53128=CARTESIAN_POINT('',(-308.,-14.0000000000001,22.));
#53129=CARTESIAN_POINT('Origin',(-308.,-14.0000000000001,25.));
#53130=CARTESIAN_POINT('',(-320.,-14.0000000000001,22.));
#53131=CARTESIAN_POINT('',(-320.,-14.0000000000001,22.));
#53132=CARTESIAN_POINT('Origin',(-320.,-14.0000000000001,25.));
#53133=CARTESIAN_POINT('Origin',(-320.,33.9999999999999,-25.));
#53134=CARTESIAN_POINT('',(-308.,33.9999999999999,-27.5));
#53135=CARTESIAN_POINT('Origin',(-308.,33.9999999999999,-25.));
#53136=CARTESIAN_POINT('',(-320.,33.9999999999999,-27.5));
#53137=CARTESIAN_POINT('',(-320.,33.9999999999999,-27.5));
#53138=CARTESIAN_POINT('Origin',(-320.,33.9999999999999,-25.));
#53139=CARTESIAN_POINT('Origin',(-320.,33.9999999999999,25.));
#53140=CARTESIAN_POINT('',(-308.,33.9999999999999,22.5));
#53141=CARTESIAN_POINT('Origin',(-308.,33.9999999999999,25.));
#53142=CARTESIAN_POINT('',(-320.,33.9999999999999,22.5));
#53143=CARTESIAN_POINT('',(-320.,33.9999999999999,22.5));
#53144=CARTESIAN_POINT('Origin',(-320.,33.9999999999999,25.));
#53145=CARTESIAN_POINT('Origin',(-320.,-34.0000000000001,25.));
#53146=CARTESIAN_POINT('',(-308.,-34.0000000000001,22.5));
#53147=CARTESIAN_POINT('Origin',(-308.,-34.0000000000001,25.));
#53148=CARTESIAN_POINT('',(-320.,-34.0000000000001,22.5));
#53149=CARTESIAN_POINT('',(-320.,-34.0000000000001,22.5));
#53150=CARTESIAN_POINT('Origin',(-320.,-34.0000000000001,25.));
#53151=CARTESIAN_POINT('Origin',(-320.,-34.0000000000001,-25.));
#53152=CARTESIAN_POINT('',(-308.,-34.0000000000001,-27.5));
#53153=CARTESIAN_POINT('Origin',(-308.,-34.0000000000001,-25.));
#53154=CARTESIAN_POINT('',(-320.,-34.0000000000001,-27.5));
#53155=CARTESIAN_POINT('',(-320.,-34.0000000000001,-27.5));
#53156=CARTESIAN_POINT('Origin',(-320.,-34.0000000000001,-25.));
#53157=CARTESIAN_POINT('Origin',(-308.,-94.,40.));
#53158=CARTESIAN_POINT('',(-314.4,-94.,45.5));
#53159=CARTESIAN_POINT('Origin',(-314.4,-94.,40.));
#53160=CARTESIAN_POINT('',(-308.,-94.,45.5));
#53161=CARTESIAN_POINT('',(-308.,-94.,45.5));
#53162=CARTESIAN_POINT('Origin',(-308.,-94.,40.));
#53163=CARTESIAN_POINT('Origin',(-308.,-94.,40.));
#53164=CARTESIAN_POINT('',(-320.,-94.,43.3));
#53165=CARTESIAN_POINT('Origin',(-320.,-94.,40.));
#53166=CARTESIAN_POINT('',(-314.4,-94.,43.3));
#53167=CARTESIAN_POINT('',(-308.,-94.,43.3));
#53168=CARTESIAN_POINT('Origin',(-314.4,-94.,40.));
#53169=CARTESIAN_POINT('Origin',(-308.,-93.9999999999999,84.9999999999999));
#53170=CARTESIAN_POINT('',(-314.4,-93.9999999999999,90.5));
#53171=CARTESIAN_POINT('Origin',(-314.4,-93.9999999999999,84.9999999999999));
#53172=CARTESIAN_POINT('',(-308.,-93.9999999999999,90.5));
#53173=CARTESIAN_POINT('',(-308.,-93.9999999999999,90.5));
#53174=CARTESIAN_POINT('Origin',(-308.,-93.9999999999999,84.9999999999999));
#53175=CARTESIAN_POINT('Origin',(-308.,-93.9999999999999,84.9999999999999));
#53176=CARTESIAN_POINT('',(-320.,-93.9999999999999,88.3));
#53177=CARTESIAN_POINT('Origin',(-320.,-93.9999999999999,84.9999999999999));
#53178=CARTESIAN_POINT('',(-314.4,-93.9999999999999,88.3));
#53179=CARTESIAN_POINT('',(-308.,-93.9999999999999,88.3));
#53180=CARTESIAN_POINT('Origin',(-314.4,-93.9999999999999,84.9999999999999));
#53181=CARTESIAN_POINT('Origin',(-308.,-151.,85.));
#53182=CARTESIAN_POINT('',(-314.4,-151.,90.5));
#53183=CARTESIAN_POINT('Origin',(-314.4,-151.,85.));
#53184=CARTESIAN_POINT('',(-308.,-151.,90.5));
#53185=CARTESIAN_POINT('',(-308.,-151.,90.5));
#53186=CARTESIAN_POINT('Origin',(-308.,-151.,85.));
#53187=CARTESIAN_POINT('Origin',(-308.,-151.,85.));
#53188=CARTESIAN_POINT('',(-320.,-151.,88.3));
#53189=CARTESIAN_POINT('Origin',(-320.,-151.,85.));
#53190=CARTESIAN_POINT('',(-314.4,-151.,88.3));
#53191=CARTESIAN_POINT('',(-308.,-151.,88.3));
#53192=CARTESIAN_POINT('Origin',(-314.4,-151.,85.));
#53193=CARTESIAN_POINT('Origin',(-308.,-151.,40.));
#53194=CARTESIAN_POINT('',(-314.4,-151.,45.5));
#53195=CARTESIAN_POINT('Origin',(-314.4,-151.,40.));
#53196=CARTESIAN_POINT('',(-308.,-151.,45.5));
#53197=CARTESIAN_POINT('',(-308.,-151.,45.5));
#53198=CARTESIAN_POINT('Origin',(-308.,-151.,40.));
#53199=CARTESIAN_POINT('Origin',(-308.,-151.,40.));
#53200=CARTESIAN_POINT('',(-320.,-151.,43.3));
#53201=CARTESIAN_POINT('Origin',(-320.,-151.,40.));
#53202=CARTESIAN_POINT('',(-314.4,-151.,43.3));
#53203=CARTESIAN_POINT('',(-308.,-151.,43.3));
#53204=CARTESIAN_POINT('Origin',(-314.4,-151.,40.));
#53205=CARTESIAN_POINT('Origin',(-308.,151.,40.));
#53206=CARTESIAN_POINT('',(-314.4,151.,45.5));
#53207=CARTESIAN_POINT('Origin',(-314.4,151.,40.));
#53208=CARTESIAN_POINT('',(-308.,151.,45.5));
#53209=CARTESIAN_POINT('',(-308.,151.,45.5));
#53210=CARTESIAN_POINT('Origin',(-308.,151.,40.));
#53211=CARTESIAN_POINT('Origin',(-308.,151.,40.));
#53212=CARTESIAN_POINT('',(-320.,151.,43.3));
#53213=CARTESIAN_POINT('Origin',(-320.,151.,40.));
#53214=CARTESIAN_POINT('',(-314.4,151.,43.3));
#53215=CARTESIAN_POINT('',(-308.,151.,43.3));
#53216=CARTESIAN_POINT('Origin',(-314.4,151.,40.));
#53217=CARTESIAN_POINT('Origin',(-308.,151.,85.));
#53218=CARTESIAN_POINT('',(-314.4,151.,90.5));
#53219=CARTESIAN_POINT('Origin',(-314.4,151.,85.));
#53220=CARTESIAN_POINT('',(-308.,151.,90.5));
#53221=CARTESIAN_POINT('',(-308.,151.,90.5));
#53222=CARTESIAN_POINT('Origin',(-308.,151.,85.));
#53223=CARTESIAN_POINT('Origin',(-308.,151.,85.));
#53224=CARTESIAN_POINT('',(-320.,151.,88.3));
#53225=CARTESIAN_POINT('Origin',(-320.,151.,85.));
#53226=CARTESIAN_POINT('',(-314.4,151.,88.3));
#53227=CARTESIAN_POINT('',(-308.,151.,88.3));
#53228=CARTESIAN_POINT('Origin',(-314.4,151.,85.));
#53229=CARTESIAN_POINT('Origin',(-308.,94.,85.));
#53230=CARTESIAN_POINT('',(-314.4,94.,90.5));
#53231=CARTESIAN_POINT('Origin',(-314.4,94.,85.));
#53232=CARTESIAN_POINT('',(-308.,94.,90.5));
#53233=CARTESIAN_POINT('',(-308.,94.,90.5));
#53234=CARTESIAN_POINT('Origin',(-308.,94.,85.));
#53235=CARTESIAN_POINT('Origin',(-308.,94.,85.));
#53236=CARTESIAN_POINT('',(-320.,94.,88.3));
#53237=CARTESIAN_POINT('Origin',(-320.,94.,85.));
#53238=CARTESIAN_POINT('',(-314.4,94.,88.3));
#53239=CARTESIAN_POINT('',(-308.,94.,88.3));
#53240=CARTESIAN_POINT('Origin',(-314.4,94.,85.));
#53241=CARTESIAN_POINT('Origin',(-308.,94.,40.));
#53242=CARTESIAN_POINT('',(-314.4,94.,45.5));
#53243=CARTESIAN_POINT('Origin',(-314.4,94.,40.));
#53244=CARTESIAN_POINT('',(-308.,94.,45.5));
#53245=CARTESIAN_POINT('',(-308.,94.,45.5));
#53246=CARTESIAN_POINT('Origin',(-308.,94.,40.));
#53247=CARTESIAN_POINT('Origin',(-308.,94.,40.));
#53248=CARTESIAN_POINT('',(-320.,94.,43.3));
#53249=CARTESIAN_POINT('Origin',(-320.,94.,40.));
#53250=CARTESIAN_POINT('',(-314.4,94.,43.3));
#53251=CARTESIAN_POINT('',(-308.,94.,43.3));
#53252=CARTESIAN_POINT('Origin',(-314.4,94.,40.));
#53253=CARTESIAN_POINT('Origin',(-308.,-94.,-85.0000000000001));
#53254=CARTESIAN_POINT('',(-314.4,-94.,-79.5));
#53255=CARTESIAN_POINT('Origin',(-314.4,-94.,-85.0000000000001));
#53256=CARTESIAN_POINT('',(-308.,-94.,-79.5));
#53257=CARTESIAN_POINT('',(-308.,-94.,-79.5));
#53258=CARTESIAN_POINT('Origin',(-308.,-94.,-85.0000000000001));
#53259=CARTESIAN_POINT('Origin',(-308.,-94.,-85.0000000000001));
#53260=CARTESIAN_POINT('',(-320.,-94.,-81.7));
#53261=CARTESIAN_POINT('Origin',(-320.,-94.,-85.0000000000001));
#53262=CARTESIAN_POINT('',(-314.4,-94.,-81.7));
#53263=CARTESIAN_POINT('',(-308.,-94.,-81.7));
#53264=CARTESIAN_POINT('Origin',(-314.4,-94.,-85.0000000000001));
#53265=CARTESIAN_POINT('Origin',(-308.,-93.9999999999999,-40.0000000000001));
#53266=CARTESIAN_POINT('',(-314.4,-93.9999999999999,-34.5000000000001));
#53267=CARTESIAN_POINT('Origin',(-314.4,-93.9999999999999,-40.0000000000001));
#53268=CARTESIAN_POINT('',(-308.,-93.9999999999999,-34.5000000000001));
#53269=CARTESIAN_POINT('',(-308.,-93.9999999999999,-34.5000000000001));
#53270=CARTESIAN_POINT('Origin',(-308.,-93.9999999999999,-40.0000000000001));
#53271=CARTESIAN_POINT('Origin',(-308.,-93.9999999999999,-40.0000000000001));
#53272=CARTESIAN_POINT('',(-320.,-93.9999999999999,-36.7));
#53273=CARTESIAN_POINT('Origin',(-320.,-93.9999999999999,-40.0000000000001));
#53274=CARTESIAN_POINT('',(-314.4,-93.9999999999999,-36.7));
#53275=CARTESIAN_POINT('',(-308.,-93.9999999999999,-36.7));
#53276=CARTESIAN_POINT('Origin',(-314.4,-93.9999999999999,-40.0000000000001));
#53277=CARTESIAN_POINT('Origin',(-308.,-151.,-40.));
#53278=CARTESIAN_POINT('',(-314.4,-151.,-34.5));
#53279=CARTESIAN_POINT('Origin',(-314.4,-151.,-40.));
#53280=CARTESIAN_POINT('',(-308.,-151.,-34.5));
#53281=CARTESIAN_POINT('',(-308.,-151.,-34.5));
#53282=CARTESIAN_POINT('Origin',(-308.,-151.,-40.));
#53283=CARTESIAN_POINT('Origin',(-308.,-151.,-40.));
#53284=CARTESIAN_POINT('',(-320.,-151.,-36.7));
#53285=CARTESIAN_POINT('Origin',(-320.,-151.,-40.));
#53286=CARTESIAN_POINT('',(-314.4,-151.,-36.7));
#53287=CARTESIAN_POINT('',(-308.,-151.,-36.7));
#53288=CARTESIAN_POINT('Origin',(-314.4,-151.,-40.));
#53289=CARTESIAN_POINT('Origin',(-308.,-151.,-85.));
#53290=CARTESIAN_POINT('',(-314.4,-151.,-79.5));
#53291=CARTESIAN_POINT('Origin',(-314.4,-151.,-85.));
#53292=CARTESIAN_POINT('',(-308.,-151.,-79.5));
#53293=CARTESIAN_POINT('',(-308.,-151.,-79.5));
#53294=CARTESIAN_POINT('Origin',(-308.,-151.,-85.));
#53295=CARTESIAN_POINT('Origin',(-308.,-151.,-85.));
#53296=CARTESIAN_POINT('',(-320.,-151.,-81.7));
#53297=CARTESIAN_POINT('Origin',(-320.,-151.,-85.));
#53298=CARTESIAN_POINT('',(-314.4,-151.,-81.7));
#53299=CARTESIAN_POINT('',(-308.,-151.,-81.7));
#53300=CARTESIAN_POINT('Origin',(-314.4,-151.,-85.));
#53301=CARTESIAN_POINT('Origin',(-308.,151.,-85.));
#53302=CARTESIAN_POINT('',(-314.4,151.,-79.5));
#53303=CARTESIAN_POINT('Origin',(-314.4,151.,-85.));
#53304=CARTESIAN_POINT('',(-308.,151.,-79.5));
#53305=CARTESIAN_POINT('',(-308.,151.,-79.5));
#53306=CARTESIAN_POINT('Origin',(-308.,151.,-85.));
#53307=CARTESIAN_POINT('Origin',(-308.,151.,-85.));
#53308=CARTESIAN_POINT('',(-320.,151.,-81.7));
#53309=CARTESIAN_POINT('Origin',(-320.,151.,-85.));
#53310=CARTESIAN_POINT('',(-314.4,151.,-81.7));
#53311=CARTESIAN_POINT('',(-308.,151.,-81.7));
#53312=CARTESIAN_POINT('Origin',(-314.4,151.,-85.));
#53313=CARTESIAN_POINT('Origin',(-308.,151.,-40.));
#53314=CARTESIAN_POINT('',(-314.4,151.,-34.5));
#53315=CARTESIAN_POINT('Origin',(-314.4,151.,-40.));
#53316=CARTESIAN_POINT('',(-308.,151.,-34.5));
#53317=CARTESIAN_POINT('',(-308.,151.,-34.5));
#53318=CARTESIAN_POINT('Origin',(-308.,151.,-40.));
#53319=CARTESIAN_POINT('Origin',(-308.,151.,-40.));
#53320=CARTESIAN_POINT('',(-320.,151.,-36.7));
#53321=CARTESIAN_POINT('Origin',(-320.,151.,-40.));
#53322=CARTESIAN_POINT('',(-314.4,151.,-36.7));
#53323=CARTESIAN_POINT('',(-308.,151.,-36.7));
#53324=CARTESIAN_POINT('Origin',(-314.4,151.,-40.));
#53325=CARTESIAN_POINT('Origin',(-308.,94.,-40.));
#53326=CARTESIAN_POINT('',(-314.4,94.,-34.5));
#53327=CARTESIAN_POINT('Origin',(-314.4,94.,-40.));
#53328=CARTESIAN_POINT('',(-308.,94.,-34.5));
#53329=CARTESIAN_POINT('',(-308.,94.,-34.5));
#53330=CARTESIAN_POINT('Origin',(-308.,94.,-40.));
#53331=CARTESIAN_POINT('Origin',(-308.,94.,-40.));
#53332=CARTESIAN_POINT('',(-320.,94.,-36.7));
#53333=CARTESIAN_POINT('Origin',(-320.,94.,-40.));
#53334=CARTESIAN_POINT('',(-314.4,94.,-36.7));
#53335=CARTESIAN_POINT('',(-308.,94.,-36.7));
#53336=CARTESIAN_POINT('Origin',(-314.4,94.,-40.));
#53337=CARTESIAN_POINT('Origin',(-308.,94.,-85.));
#53338=CARTESIAN_POINT('',(-314.4,94.,-79.5));
#53339=CARTESIAN_POINT('Origin',(-314.4,94.,-85.));
#53340=CARTESIAN_POINT('',(-308.,94.,-79.5));
#53341=CARTESIAN_POINT('',(-308.,94.,-79.5));
#53342=CARTESIAN_POINT('Origin',(-308.,94.,-85.));
#53343=CARTESIAN_POINT('Origin',(-308.,94.,-85.));
#53344=CARTESIAN_POINT('',(-320.,94.,-81.7));
#53345=CARTESIAN_POINT('Origin',(-320.,94.,-85.));
#53346=CARTESIAN_POINT('',(-314.4,94.,-81.7));
#53347=CARTESIAN_POINT('',(-308.,94.,-81.7));
#53348=CARTESIAN_POINT('Origin',(-314.4,94.,-85.));
#53349=CARTESIAN_POINT('Origin',(-320.,-160.,6.));
#53350=CARTESIAN_POINT('',(-320.,-155.,-110.));
#53351=CARTESIAN_POINT('',(-320.,155.,-110.));
#53352=CARTESIAN_POINT('',(-320.,175.,-110.));
#53353=CARTESIAN_POINT('',(-320.,-175.,-89.9999999999999));
#53354=CARTESIAN_POINT('',(-320.,-215.5,-49.4999999999997));
#53355=CARTESIAN_POINT('',(-320.,-175.,90.));
#53356=CARTESIAN_POINT('',(-320.,-175.,110.));
#53357=CARTESIAN_POINT('',(-320.,-155.,110.));
#53358=CARTESIAN_POINT('',(-320.,-209.5,55.5000000000003));
#53359=CARTESIAN_POINT('',(-320.,155.,110.));
#53360=CARTESIAN_POINT('',(-320.,175.,110.));
#53361=CARTESIAN_POINT('',(-320.,175.,89.9999999999999));
#53362=CARTESIAN_POINT('',(-320.,49.5000000000005,215.5));
#53363=CARTESIAN_POINT('',(-320.,175.,-90.));
#53364=CARTESIAN_POINT('',(-320.,175.,110.));
#53365=CARTESIAN_POINT('',(-320.,55.499999999999,-209.5));
#53366=CARTESIAN_POINT('Origin',(-320.,-160.,6.));
#53367=CARTESIAN_POINT('',(-308.,-160.,-6.));
#53368=CARTESIAN_POINT('',(64.9999999999998,-160.,-6.));
#53369=CARTESIAN_POINT('',(-320.,-160.,-6.));
#53370=CARTESIAN_POINT('',(64.9999999999998,-160.,6.));
#53371=CARTESIAN_POINT('',(64.9999999999999,-160.,6.));
#53372=CARTESIAN_POINT('',(-308.,-160.,6.));
#53373=CARTESIAN_POINT('',(-320.,-160.,6.));
#53374=CARTESIAN_POINT('',(-308.,-160.,6.));
#53375=CARTESIAN_POINT('Origin',(115.,-160.,6.));
#53376=CARTESIAN_POINT('',(115.,-110.,6.));
#53377=CARTESIAN_POINT('',(115.,110.,6.));
#53378=CARTESIAN_POINT('',(115.,-160.,6.));
#53379=CARTESIAN_POINT('',(115.,-110.,-6.));
#53380=CARTESIAN_POINT('',(115.,-110.,6.));
#53381=CARTESIAN_POINT('',(115.,110.,-6.));
#53382=CARTESIAN_POINT('',(115.,-160.,-6.));
#53383=CARTESIAN_POINT('',(115.,110.,6.));
#53384=CARTESIAN_POINT('Origin',(-320.,160.,6.));
#53385=CARTESIAN_POINT('',(-308.,160.,6.));
#53386=CARTESIAN_POINT('',(64.9999999999999,160.,6.));
#53387=CARTESIAN_POINT('',(-320.,160.,6.));
#53388=CARTESIAN_POINT('',(64.9999999999999,160.,-6.));
#53389=CARTESIAN_POINT('',(64.9999999999999,160.,-6.));
#53390=CARTESIAN_POINT('',(-308.,160.,-6.));
#53391=CARTESIAN_POINT('',(-320.,160.,-6.));
#53392=CARTESIAN_POINT('',(-308.,160.,6.));
#53393=CARTESIAN_POINT('Origin',(0.,0.,6.));
#53394=CARTESIAN_POINT('',(115.,-110.,6.));
#53395=CARTESIAN_POINT('',(64.9999999999999,160.,6.));
#53396=CARTESIAN_POINT('',(-308.,0.,6.));
#53397=CARTESIAN_POINT('',(17.5,-55.,6.00000000000001));
#53398=CARTESIAN_POINT('',(17.5,-55.,6.00000000000001));
#53399=CARTESIAN_POINT('',(17.5,55.,6.00000000000001));
#53400=CARTESIAN_POINT('',(17.5,55.,6.00000000000001));
#53401=CARTESIAN_POINT('Origin',(17.5,0.,6.00000000000001));
#53402=CARTESIAN_POINT('Origin',(0.,0.,-6.));
#53403=CARTESIAN_POINT('',(112.5,-112.5,-6.));
#53404=CARTESIAN_POINT('',(-308.,0.,-6.));
#53405=CARTESIAN_POINT('',(112.5,112.5,-6.));
#53406=CARTESIAN_POINT('',(17.5,-55.,-6.));
#53407=CARTESIAN_POINT('',(17.5,-55.,-6.));
#53408=CARTESIAN_POINT('',(17.5,55.,-6.));
#53409=CARTESIAN_POINT('Origin',(17.5,0.,-6.));
#53410=CARTESIAN_POINT('',(17.5,55.,-6.));
#53411=CARTESIAN_POINT('Origin',(-308.,0.,0.));
#53412=CARTESIAN_POINT('',(-308.,-175.,90.));
#53413=CARTESIAN_POINT('',(-308.,-175.,-89.9999999999999));
#53414=CARTESIAN_POINT('',(-308.,-175.,110.));
#53415=CARTESIAN_POINT('',(-308.,-155.,-110.));
#53416=CARTESIAN_POINT('',(-308.,-132.5,-132.5));
#53417=CARTESIAN_POINT('',(-308.,155.,-110.));
#53418=CARTESIAN_POINT('',(-308.,175.,-110.));
#53419=CARTESIAN_POINT('',(-308.,175.,-90.));
#53420=CARTESIAN_POINT('',(-308.,132.499999999999,-132.5));
#53421=CARTESIAN_POINT('',(-308.,175.,89.9999999999999));
#53422=CARTESIAN_POINT('',(-308.,175.,110.));
#53423=CARTESIAN_POINT('',(-308.,155.,110.));
#53424=CARTESIAN_POINT('',(-308.,132.5,132.5));
#53425=CARTESIAN_POINT('',(-308.,-155.,110.));
#53426=CARTESIAN_POINT('',(-308.,175.,110.));
#53427=CARTESIAN_POINT('',(-308.,-132.499999999999,132.5));
#53428=CARTESIAN_POINT('Origin',(-308.,175.,-110.));
#53429=CARTESIAN_POINT('',(-308.,-155.,-110.));
#53430=CARTESIAN_POINT('',(-308.,155.,-110.));
#53431=CARTESIAN_POINT('Origin',(-308.,175.,110.));
#53432=CARTESIAN_POINT('',(-308.,175.,89.9999999999999));
#53433=CARTESIAN_POINT('',(-308.,175.,-90.));
#53434=CARTESIAN_POINT('Origin',(-308.,175.,110.));
#53435=CARTESIAN_POINT('',(-308.,-155.,110.));
#53436=CARTESIAN_POINT('',(-308.,155.,110.));
#53437=CARTESIAN_POINT('Origin',(-308.,-175.,110.));
#53438=CARTESIAN_POINT('',(-308.,-175.,-89.9999999999999));
#53439=CARTESIAN_POINT('',(-308.,-175.,90.));
#53440=CARTESIAN_POINT('Origin',(-314.4,97.3,-85.));
#53441=CARTESIAN_POINT('Origin',(-314.4,97.3,-40.));
#53442=CARTESIAN_POINT('Origin',(-314.4,154.3,-40.));
#53443=CARTESIAN_POINT('Origin',(-314.4,154.3,-85.));
#53444=CARTESIAN_POINT('Origin',(-314.4,-147.7,-85.));
#53445=CARTESIAN_POINT('Origin',(-314.4,-147.7,-40.));
#53446=CARTESIAN_POINT('Origin',(-314.4,-90.6999999999999,-40.0000000000001));
#53447=CARTESIAN_POINT('Origin',(-314.4,-90.7,-85.0000000000001));
#53448=CARTESIAN_POINT('Origin',(-314.4,97.3,40.));
#53449=CARTESIAN_POINT('Origin',(-314.4,97.3,85.));
#53450=CARTESIAN_POINT('Origin',(-314.4,154.3,85.));
#53451=CARTESIAN_POINT('Origin',(-314.4,154.3,40.));
#53452=CARTESIAN_POINT('Origin',(-314.4,-147.7,40.));
#53453=CARTESIAN_POINT('Origin',(-314.4,-147.7,85.));
#53454=CARTESIAN_POINT('Origin',(-314.4,-90.6999999999999,84.9999999999999));
#53455=CARTESIAN_POINT('Origin',(-314.4,-90.7,40.));
#53456=CARTESIAN_POINT('Origin',(-190.,0.,1.));
#53457=CARTESIAN_POINT('Origin',(115.,-110.,6.));
#53458=CARTESIAN_POINT('Origin',(64.9999999999999,160.,6.));
#53459=CARTESIAN_POINT('Origin',(17.5,-55.,110.001));
#53460=CARTESIAN_POINT('',(17.5,-55.,110.001));
#53461=CARTESIAN_POINT('Origin',(17.5,55.,110.001));
#53462=CARTESIAN_POINT('',(17.5,55.,110.001));
#53463=CARTESIAN_POINT('Origin',(17.5,0.,110.001));
#53464=CARTESIAN_POINT('Origin',(-308.,-155.,-110.));
#53465=CARTESIAN_POINT('Origin',(-308.,-175.,90.));
#53466=CARTESIAN_POINT('Origin',(-308.,155.,110.));
#53467=CARTESIAN_POINT('Origin',(-308.,175.,-90.));
#57029=UNCERTAINTY_MEASURE_WITH_UNIT(LENGTH_MEASURE(0.01),#57080,
'DISTANCE_ACCURACY_VALUE',
'Maximum model space distance between geometric entities at asserted c
onnectivities');
#57040=UNCERTAINTY_MEASURE_WITH_UNIT(LENGTH_MEASURE(0.01),#57080,
'DISTANCE_ACCURACY_VALUE',
'Maximum model space distance between geometric entities at asserted c
onnectivities');
#57068=(
GEOMETRIC_REPRESENTATION_CONTEXT(3)
GLOBAL_UNCERTAINTY_ASSIGNED_CONTEXT((#57029))
GLOBAL_UNIT_ASSIGNED_CONTEXT((#57080,#57082,#57083))
REPRESENTATION_CONTEXT('','3D')
);
#57079=(
GEOMETRIC_REPRESENTATION_CONTEXT(3)
GLOBAL_UNCERTAINTY_ASSIGNED_CONTEXT((#57040))
GLOBAL_UNIT_ASSIGNED_CONTEXT((#57080,#57082,#57083))
REPRESENTATION_CONTEXT('','3D')
);
#57080=(
LENGTH_UNIT()
NAMED_UNIT(*)
SI_UNIT(.MILLI.,.METRE.)
);
#57082=(
NAMED_UNIT(*)
PLANE_ANGLE_UNIT()
SI_UNIT($,.RADIAN.)
);
#57083=(
NAMED_UNIT(*)
SI_UNIT($,.STERADIAN.)
SOLID_ANGLE_UNIT()
);
#57111=SHAPE_DEFINITION_REPRESENTATION(#57165,#57276);
#57165=PRODUCT_DEFINITION_SHAPE('',$,#57315);
#57276=SHAPE_REPRESENTATION('',(#26068),#57068);
#57287=PRODUCT_DEFINITION_CONTEXT('part definition',#57403,'design');
#57315=PRODUCT_DEFINITION('Motor Mount Bracket','Motor Mount Bracket',#57353,
#57287);
#57353=PRODUCT_DEFINITION_FORMATION('',$,#57432);
#57403=APPLICATION_CONTEXT(
'Core Data for Automotive Mechanical Design Process');
#57404=PRODUCT_CONTEXT('part definition',#57403,'mechanical');
#57432=PRODUCT('Motor Mount Bracket','Motor Mount Bracket',$,(#57404));
#57444=PRESENTATION_STYLE_ASSIGNMENT((#57446));
#57446=SURFACE_STYLE_USAGE(.BOTH.,#57448);
#57448=SURFACE_SIDE_STYLE('',(#57450));
#57450=SURFACE_STYLE_FILL_AREA(#57452);
#57452=FILL_AREA_STYLE('Opaque(202,209,238)',(#57454));
#57454=FILL_AREA_STYLE_COLOUR('Opaque(202,209,238)',#57456);
#57456=COLOUR_RGB('Opaque(202,209,238)',0.792156862745098,0.819607843137255,
0.933333333333333);
ENDSEC;
END-ISO-10303-21;
